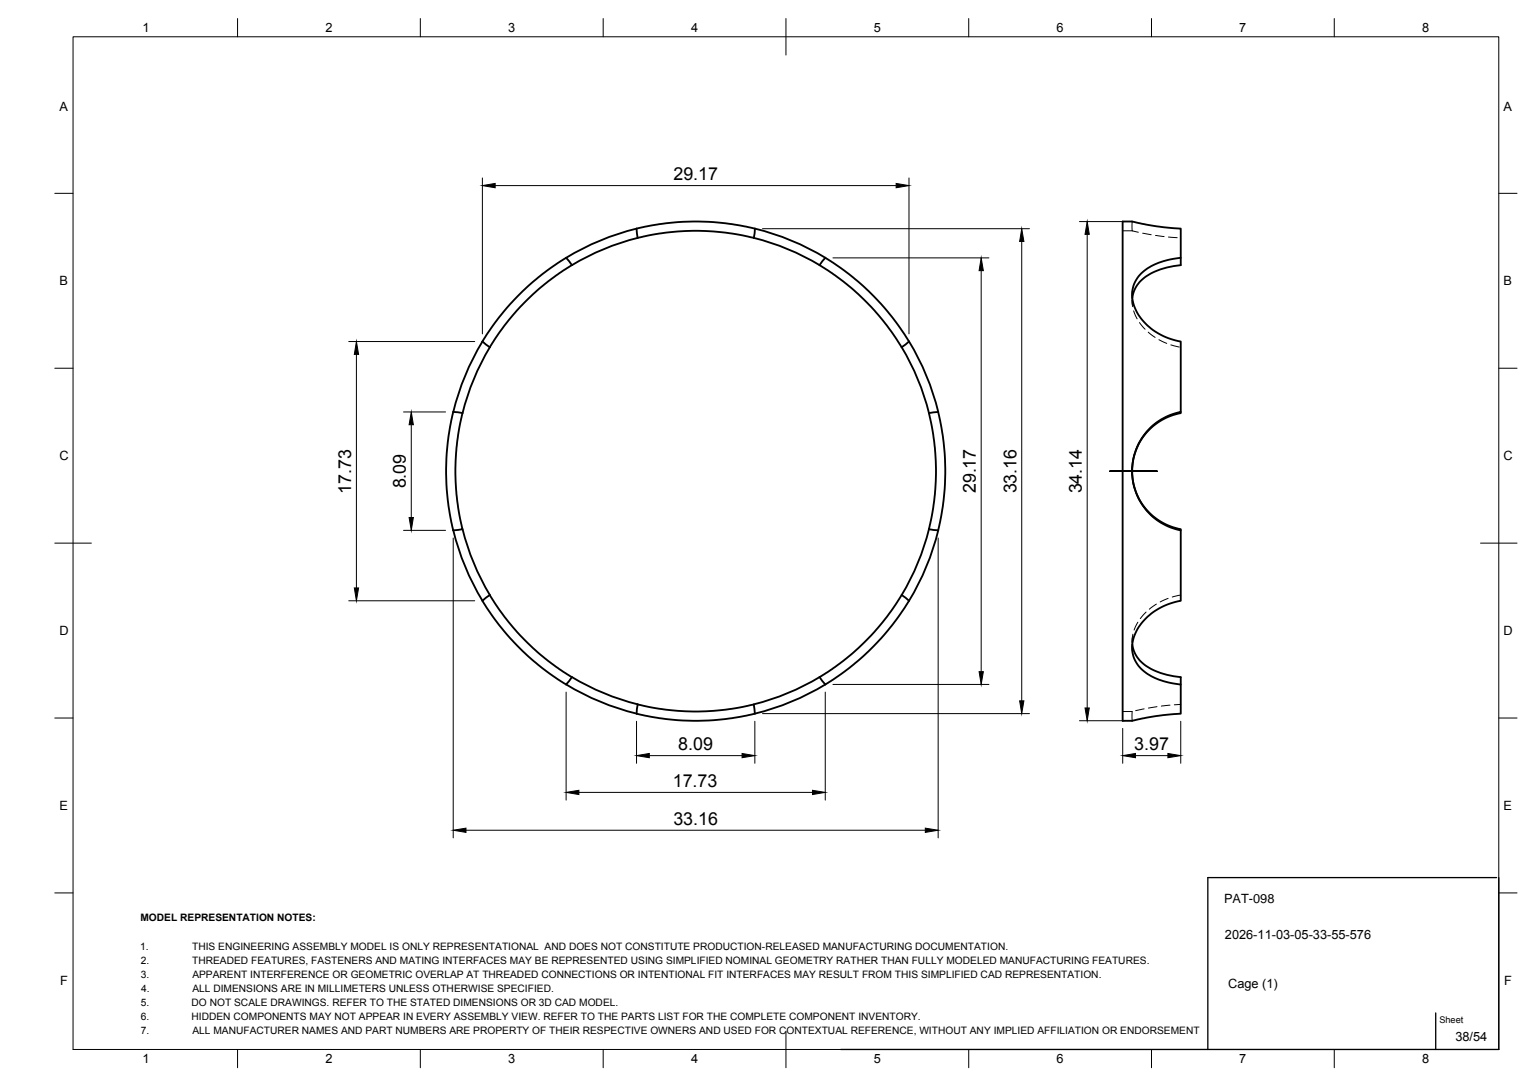
ISO-10303-21;
HEADER;
/* Generated by software containing ST-Developer
 * from STEP Tools, Inc. (www.steptools.com) 
 */

FILE_DESCRIPTION(
/* description */ ('Spring compression tester'),
/* implementation_level */ '2;1');

FILE_NAME(
/* name */ 'Cage (1).step',
/* time_stamp */ '2026-10-28T03:24:11-07:00',
/* author */ (''),
/* organization */ (''),
/* preprocessor_version */ 'ST-DEVELOPER v20.2',
/* originating_system */ 'Autodesk Translation Framework v15.17.0.0',
/* authorisation */ '');

FILE_SCHEMA (('AUTOMOTIVE_DESIGN { 1 0 10303 214 3 1 1 }'));
ENDSEC;

DATA;
#10=MECHANICAL_DESIGN_GEOMETRIC_PRESENTATION_REPRESENTATION('',(#1149),#43521);
#567=B_SPLINE_CURVE_WITH_KNOTS('',3,(#29122,#29123,#29124,#29125,#29126,
#29127,#29128,#29129,#29130,#29131,#29132,#29133,#29134,#29135,#29136,#29137,
#29138,#29139,#29140,#29141,#29142,#29143),.UNSPECIFIED.,.F.,.F.,(4,2,2,
2,2,2,2,2,2,2,4),(0.0789094028588958,0.210573405340968,0.315860108011452,
0.421146810681936,0.522142632548711,0.623138454415485,0.72413427628226,
0.825130098149035,0.930416800819519,1.03570350349,1.16736750597208),
 .UNSPECIFIED.);
#568=B_SPLINE_CURVE_WITH_KNOTS('',3,(#29147,#29148,#29149,#29150,#29151,
#29152,#29153,#29154,#29155,#29156,#29157,#29158,#29159,#29160,#29161,#29162,
#29163,#29164,#29165,#29166,#29167,#29168),.UNSPECIFIED.,.F.,.F.,(4,2,2,
2,2,2,2,2,2,2,4),(0.0774793363974613,0.142088896491891,0.284177792983782,
0.411119756996526,0.514392970548519,0.617666184100513,0.720939397652506,
0.8242126112045,0.951154575217244,1.09324347170913,1.15785303180356),
 .UNSPECIFIED.);
#569=B_SPLINE_CURVE_WITH_KNOTS('',3,(#29174,#29175,#29176,#29177,#29178,
#29179,#29180,#29181,#29182,#29183,#29184,#29185,#29186,#29187,#29188,#29189,
#29190,#29191,#29192,#29193,#29194,#29195),.UNSPECIFIED.,.F.,.F.,(4,2,2,
2,2,2,2,2,2,2,4),(0.0774793363974613,0.142088896491891,0.284177792983782,
0.411119756996525,0.514392970548519,0.617666184100513,0.720939397652506,
0.8242126112045,0.951154575217243,1.09324347170913,1.15785303180356),
 .UNSPECIFIED.);
#570=B_SPLINE_CURVE_WITH_KNOTS('',3,(#29199,#29200,#29201,#29202,#29203,
#29204,#29205,#29206,#29207,#29208,#29209,#29210,#29211,#29212,#29213,#29214,
#29215,#29216,#29217,#29218,#29219,#29220),.UNSPECIFIED.,.F.,.F.,(4,2,2,
2,2,2,2,2,2,2,4),(0.0774793363974614,0.142088896491891,0.284177792983781,
0.411119756996525,0.514392970548519,0.617666184100512,0.720939397652506,
0.824212611204499,0.951154575217243,1.09324347170913,1.15785303180356),
 .UNSPECIFIED.);
#571=B_SPLINE_CURVE_WITH_KNOTS('',3,(#29224,#29225,#29226,#29227,#29228,
#29229,#29230,#29231,#29232,#29233,#29234,#29235),.UNSPECIFIED.,.F.,.F.,
(4,2,2,2,2,4),(0.0774793363974613,0.142088896491891,0.284177792983781,0.411119756996525,
0.514392970548519,0.617666184100512),.UNSPECIFIED.);
#572=B_SPLINE_CURVE_WITH_KNOTS('',3,(#29240,#29241,#29242,#29243,#29244,
#29245,#29246,#29247,#29248,#29249,#29250,#29251),.UNSPECIFIED.,.F.,.F.,
(4,2,2,2,2,4),(0.617666184100512,0.720939397652506,0.824212611204499,0.951154575217243,
1.09324347170913,1.15785303180356),.UNSPECIFIED.);
#573=B_SPLINE_CURVE_WITH_KNOTS('',3,(#29255,#29256,#29257,#29258,#29259,
#29260,#29261,#29262,#29263,#29264,#29265,#29266,#29267,#29268,#29269,#29270,
#29271,#29272,#29273,#29274,#29275,#29276),.UNSPECIFIED.,.F.,.F.,(4,2,2,
2,2,2,2,2,2,2,4),(0.0774793363974613,0.142088896491891,0.284177792983782,
0.411119756996526,0.514392970548519,0.617666184100513,0.720939397652507,
0.8242126112045,0.951154575217245,1.09324347170914,1.15785303180356),
 .UNSPECIFIED.);
#574=B_SPLINE_CURVE_WITH_KNOTS('',3,(#29280,#29281,#29282,#29283,#29284,
#29285,#29286,#29287,#29288,#29289,#29290,#29291,#29292,#29293,#29294,#29295,
#29296,#29297,#29298,#29299,#29300,#29301),.UNSPECIFIED.,.F.,.F.,(4,2,2,
2,2,2,2,2,2,2,4),(0.0774793363974613,0.142088896491891,0.284177792983782,
0.411119756996526,0.514392970548519,0.617666184100513,0.720939397652506,
0.824212611204499,0.951154575217243,1.09324347170913,1.15785303180356),
 .UNSPECIFIED.);
#575=B_SPLINE_CURVE_WITH_KNOTS('',3,(#29305,#29306,#29307,#29308,#29309,
#29310,#29311,#29312,#29313,#29314,#29315,#29316,#29317,#29318,#29319,#29320,
#29321,#29322,#29323,#29324,#29325,#29326),.UNSPECIFIED.,.F.,.F.,(4,2,2,
2,2,2,2,2,2,2,4),(0.0774793363974613,0.142088896491891,0.284177792983782,
0.411119756996526,0.514392970548519,0.617666184100513,0.720939397652506,
0.8242126112045,0.951154575217244,1.09324347170913,1.15785303180356),
 .UNSPECIFIED.);
#576=B_SPLINE_CURVE_WITH_KNOTS('',3,(#29330,#29331,#29332,#29333,#29334,
#29335,#29336,#29337,#29338,#29339,#29340,#29341,#29342,#29343,#29344,#29345,
#29346,#29347,#29348,#29349,#29350,#29351),.UNSPECIFIED.,.F.,.F.,(4,2,2,
2,2,2,2,2,2,2,4),(0.0774793363974613,0.142088896491891,0.284177792983782,
0.411119756996526,0.514392970548519,0.617666184100513,0.720939397652506,
0.8242126112045,0.951154575217243,1.09324347170913,1.15785303180356),
 .UNSPECIFIED.);
#577=B_SPLINE_CURVE_WITH_KNOTS('',3,(#29359,#29360,#29361,#29362,#29363,
#29364,#29365,#29366,#29367,#29368,#29369,#29370,#29371,#29372,#29373,#29374,
#29375,#29376,#29377,#29378,#29379,#29380),.UNSPECIFIED.,.F.,.F.,(4,2,2,
2,2,2,2,2,2,2,4),(0.0789094028588958,0.210573405340968,0.315860108011452,
0.421146810681936,0.522142632548711,0.623138454415485,0.72413427628226,
0.825130098149035,0.930416800819519,1.03570350349,1.16736750597208),
 .UNSPECIFIED.);
#578=B_SPLINE_CURVE_WITH_KNOTS('',3,(#29388,#29389,#29390,#29391,#29392,
#29393,#29394,#29395,#29396,#29397,#29398,#29399,#29400,#29401,#29402,#29403,
#29404,#29405,#29406,#29407,#29408,#29409),.UNSPECIFIED.,.F.,.F.,(4,2,2,
2,2,2,2,2,2,2,4),(0.0789094028588958,0.210573405340969,0.315860108011453,
0.421146810681937,0.522142632548712,0.623138454415486,0.724134276282261,
0.825130098149035,0.930416800819519,1.03570350349,1.16736750597208),
 .UNSPECIFIED.);
#579=B_SPLINE_CURVE_WITH_KNOTS('',3,(#29418,#29419,#29420,#29421,#29422,
#29423,#29424,#29425,#29426,#29427,#29428,#29429),.UNSPECIFIED.,.F.,.F.,
(4,2,2,2,2,4),(0.0789094028588958,0.210573405340968,0.315860108011452,0.421146810681937,
0.522142632548711,0.623138454415486),.UNSPECIFIED.);
#580=B_SPLINE_CURVE_WITH_KNOTS('',3,(#29431,#29432,#29433,#29434,#29435,
#29436,#29437,#29438,#29439,#29440,#29441,#29442),.UNSPECIFIED.,.F.,.F.,
(4,2,2,2,2,4),(0.623138454415486,0.72413427628226,0.825130098149035,0.930416800819519,
1.03570350349,1.16736750597208),.UNSPECIFIED.);
#581=B_SPLINE_CURVE_WITH_KNOTS('',3,(#29449,#29450,#29451,#29452,#29453,
#29454,#29455,#29456,#29457,#29458,#29459,#29460,#29461,#29462,#29463,#29464,
#29465,#29466,#29467,#29468,#29469,#29470),.UNSPECIFIED.,.F.,.F.,(4,2,2,
2,2,2,2,2,2,2,4),(0.0789094028588958,0.210573405340968,0.315860108011452,
0.421146810681936,0.522142632548711,0.623138454415486,0.72413427628226,
0.825130098149035,0.930416800819519,1.03570350349,1.16736750597208),
 .UNSPECIFIED.);
#582=B_SPLINE_CURVE_WITH_KNOTS('',3,(#29478,#29479,#29480,#29481,#29482,
#29483,#29484,#29485,#29486,#29487,#29488,#29489,#29490,#29491,#29492,#29493,
#29494,#29495,#29496,#29497,#29498,#29499),.UNSPECIFIED.,.F.,.F.,(4,2,2,
2,2,2,2,2,2,2,4),(0.0789094028588957,0.210573405340968,0.315860108011452,
0.421146810681936,0.522142632548711,0.623138454415485,0.72413427628226,
0.825130098149035,0.930416800819519,1.03570350349,1.16736750597207),
 .UNSPECIFIED.);
#583=B_SPLINE_CURVE_WITH_KNOTS('',3,(#29507,#29508,#29509,#29510,#29511,
#29512,#29513,#29514,#29515,#29516,#29517,#29518,#29519,#29520,#29521,#29522,
#29523,#29524,#29525,#29526,#29527,#29528),.UNSPECIFIED.,.F.,.F.,(4,2,2,
2,2,2,2,2,2,2,4),(0.0789094028588958,0.210573405340968,0.315860108011452,
0.421146810681936,0.522142632548711,0.623138454415486,0.72413427628226,
0.825130098149035,0.930416800819519,1.03570350349,1.16736750597208),
 .UNSPECIFIED.);
#584=B_SPLINE_CURVE_WITH_KNOTS('',3,(#29537,#29538,#29539,#29540,#29541,
#29542,#29543,#29544,#29545,#29546,#29547,#29548,#29549,#29550,#29551,#29552,
#29553,#29554,#29555,#29556,#29557,#29558),.UNSPECIFIED.,.F.,.F.,(4,2,2,
2,2,2,2,2,2,2,4),(0.0789094028588958,0.210573405340968,0.315860108011452,
0.421146810681936,0.522142632548711,0.623138454415485,0.72413427628226,
0.825130098149035,0.930416800819519,1.03570350349,1.16736750597208),
 .UNSPECIFIED.);
#919=SPHERICAL_SURFACE('',#20179,0.412776);
#920=SPHERICAL_SURFACE('',#20195,0.412776);
#921=SPHERICAL_SURFACE('',#20200,0.412776);
#922=SPHERICAL_SURFACE('',#20205,0.412776);
#923=SPHERICAL_SURFACE('',#20210,0.412776);
#924=SPHERICAL_SURFACE('',#20215,0.412776);
#925=SPHERICAL_SURFACE('',#20220,0.412776);
#926=SPHERICAL_SURFACE('',#20228,0.412776);
#1015=SHAPE_REPRESENTATION_RELATIONSHIP('SRR','None',#43829,#1075);
#1075=ADVANCED_BREP_SHAPE_REPRESENTATION('',(#1223),#43489);
#1149=STYLED_ITEM('',(#44202),#1223);
#1223=MANIFOLD_SOLID_BREP('Continuous crown cage',#18587);
#1463=FACE_BOUND('',#3949,.T.);
#1908=PLANE('',#20192);
#1909=PLANE('',#20197);
#1910=PLANE('',#20202);
#1911=PLANE('',#20207);
#1912=PLANE('',#20212);
#1913=PLANE('',#20217);
#1914=PLANE('',#20226);
#1915=PLANE('',#20230);
#1916=PLANE('',#20231);
#2668=FACE_OUTER_BOUND('',#3931,.T.);
#2669=FACE_OUTER_BOUND('',#3932,.T.);
#2670=FACE_OUTER_BOUND('',#3933,.T.);
#2671=FACE_OUTER_BOUND('',#3934,.T.);
#2672=FACE_OUTER_BOUND('',#3935,.T.);
#2673=FACE_OUTER_BOUND('',#3936,.T.);
#2674=FACE_OUTER_BOUND('',#3937,.T.);
#2675=FACE_OUTER_BOUND('',#3938,.T.);
#2676=FACE_OUTER_BOUND('',#3939,.T.);
#2677=FACE_OUTER_BOUND('',#3940,.T.);
#2678=FACE_OUTER_BOUND('',#3941,.T.);
#2679=FACE_OUTER_BOUND('',#3942,.T.);
#2680=FACE_OUTER_BOUND('',#3943,.T.);
#2681=FACE_OUTER_BOUND('',#3944,.T.);
#2682=FACE_OUTER_BOUND('',#3945,.T.);
#2683=FACE_OUTER_BOUND('',#3946,.T.);
#2684=FACE_OUTER_BOUND('',#3947,.T.);
#2685=FACE_OUTER_BOUND('',#3948,.T.);
#2686=FACE_OUTER_BOUND('',#3950,.T.);
#3931=EDGE_LOOP('',(#14399,#14400,#14401,#14402));
#3932=EDGE_LOOP('',(#14403,#14404,#14405,#14406,#14407,#14408,#14409,#14410,
#14411,#14412,#14413,#14414,#14415,#14416,#14417,#14418,#14419,#14420,#14421,
#14422));
#3933=EDGE_LOOP('',(#14423,#14424,#14425,#14426));
#3934=EDGE_LOOP('',(#14427,#14428,#14429,#14430));
#3935=EDGE_LOOP('',(#14431,#14432,#14433,#14434));
#3936=EDGE_LOOP('',(#14435,#14436,#14437,#14438));
#3937=EDGE_LOOP('',(#14439,#14440,#14441,#14442));
#3938=EDGE_LOOP('',(#14443,#14444,#14445,#14446,#14447,#14448));
#3939=EDGE_LOOP('',(#14449,#14450,#14451,#14452));
#3940=EDGE_LOOP('',(#14453,#14454,#14455,#14456));
#3941=EDGE_LOOP('',(#14457,#14458,#14459,#14460));
#3942=EDGE_LOOP('',(#14461,#14462,#14463,#14464));
#3943=EDGE_LOOP('',(#14465,#14466,#14467,#14468));
#3944=EDGE_LOOP('',(#14469,#14470,#14471,#14472));
#3945=EDGE_LOOP('',(#14473,#14474,#14475,#14476,#14477,#14478,#14479,#14480,
#14481,#14482,#14483,#14484,#14485,#14486,#14487,#14488,#14489,#14490,#14491,
#14492));
#3946=EDGE_LOOP('',(#14493,#14494,#14495,#14496));
#3947=EDGE_LOOP('',(#14497,#14498,#14499,#14500));
#3948=EDGE_LOOP('',(#14501));
#3949=EDGE_LOOP('',(#14502));
#3950=EDGE_LOOP('',(#14503,#14504,#14505,#14506));
#5327=LINE('',#29237,#6759);
#5328=LINE('',#29533,#6760);
#6759=VECTOR('',#23721,1.706752);
#6760=VECTOR('',#23798,1.643248);
#7826=CIRCLE('',#20180,0.405071403305639);
#7827=CIRCLE('',#20181,0.405071403305639);
#7828=CIRCLE('',#20183,1.706752);
#7829=CIRCLE('',#20184,1.706752);
#7830=CIRCLE('',#20185,1.706752);
#7831=CIRCLE('',#20186,1.706752);
#7832=CIRCLE('',#20187,1.706752);
#7833=CIRCLE('',#20188,1.706752);
#7834=CIRCLE('',#20189,1.706752);
#7835=CIRCLE('',#20190,1.706752);
#7836=CIRCLE('',#20191,1.706752);
#7837=CIRCLE('',#20193,1.643248);
#7838=CIRCLE('',#20194,0.405071403305639);
#7839=CIRCLE('',#20196,0.405071403305639);
#7840=CIRCLE('',#20198,1.643248);
#7841=CIRCLE('',#20199,0.405071403305639);
#7842=CIRCLE('',#20201,0.405071403305639);
#7843=CIRCLE('',#20203,1.643248);
#7844=CIRCLE('',#20204,0.405071403305639);
#7845=CIRCLE('',#20206,0.405071403305639);
#7846=CIRCLE('',#20208,1.643248);
#7847=CIRCLE('',#20209,0.405071403305639);
#7848=CIRCLE('',#20211,0.405071403305639);
#7849=CIRCLE('',#20213,1.643248);
#7850=CIRCLE('',#20214,0.405071403305639);
#7851=CIRCLE('',#20216,0.405071403305639);
#7852=CIRCLE('',#20218,1.643248);
#7853=CIRCLE('',#20219,0.405071403305639);
#7854=CIRCLE('',#20221,0.405071403305639);
#7855=CIRCLE('',#20223,1.643248);
#7856=CIRCLE('',#20224,1.643248);
#7857=CIRCLE('',#20225,1.643248);
#7858=CIRCLE('',#20227,0.405071403305639);
#7859=CIRCLE('',#20229,0.405071403305639);
#8879=VERTEX_POINT('',#29120);
#8880=VERTEX_POINT('',#29121);
#8881=VERTEX_POINT('',#29144);
#8882=VERTEX_POINT('',#29146);
#8883=VERTEX_POINT('',#29171);
#8884=VERTEX_POINT('',#29173);
#8885=VERTEX_POINT('',#29196);
#8886=VERTEX_POINT('',#29198);
#8887=VERTEX_POINT('',#29221);
#8888=VERTEX_POINT('',#29223);
#8889=VERTEX_POINT('',#29236);
#8890=VERTEX_POINT('',#29239);
#8891=VERTEX_POINT('',#29252);
#8892=VERTEX_POINT('',#29254);
#8893=VERTEX_POINT('',#29277);
#8894=VERTEX_POINT('',#29279);
#8895=VERTEX_POINT('',#29302);
#8896=VERTEX_POINT('',#29304);
#8897=VERTEX_POINT('',#29327);
#8898=VERTEX_POINT('',#29329);
#8899=VERTEX_POINT('',#29354);
#8900=VERTEX_POINT('',#29358);
#8901=VERTEX_POINT('',#29383);
#8902=VERTEX_POINT('',#29387);
#8903=VERTEX_POINT('',#29412);
#8904=VERTEX_POINT('',#29416);
#8905=VERTEX_POINT('',#29417);
#8906=VERTEX_POINT('',#29444);
#8907=VERTEX_POINT('',#29448);
#8908=VERTEX_POINT('',#29473);
#8909=VERTEX_POINT('',#29477);
#8910=VERTEX_POINT('',#29502);
#8911=VERTEX_POINT('',#29506);
#8912=VERTEX_POINT('',#29531);
#8913=VERTEX_POINT('',#29534);
#8914=VERTEX_POINT('',#29536);
#10864=EDGE_CURVE('',#8879,#8880,#567,.T.);
#10865=EDGE_CURVE('',#8881,#8879,#7826,.T.);
#10866=EDGE_CURVE('',#8882,#8881,#568,.T.);
#10867=EDGE_CURVE('',#8880,#8882,#7827,.T.);
#10868=EDGE_CURVE('',#8883,#8881,#7828,.T.);
#10869=EDGE_CURVE('',#8883,#8884,#569,.T.);
#10870=EDGE_CURVE('',#8885,#8884,#7829,.T.);
#10871=EDGE_CURVE('',#8885,#8886,#570,.T.);
#10872=EDGE_CURVE('',#8887,#8886,#7830,.T.);
#10873=EDGE_CURVE('',#8887,#8888,#571,.T.);
#10874=EDGE_CURVE('',#8888,#8889,#5327,.T.);
#10875=EDGE_CURVE('',#8889,#8889,#7831,.T.);
#10876=EDGE_CURVE('',#8888,#8890,#572,.T.);
#10877=EDGE_CURVE('',#8891,#8890,#7832,.T.);
#10878=EDGE_CURVE('',#8891,#8892,#573,.T.);
#10879=EDGE_CURVE('',#8893,#8892,#7833,.T.);
#10880=EDGE_CURVE('',#8893,#8894,#574,.T.);
#10881=EDGE_CURVE('',#8895,#8894,#7834,.T.);
#10882=EDGE_CURVE('',#8895,#8896,#575,.T.);
#10883=EDGE_CURVE('',#8897,#8896,#7835,.T.);
#10884=EDGE_CURVE('',#8897,#8898,#576,.T.);
#10885=EDGE_CURVE('',#8882,#8898,#7836,.T.);
#10886=EDGE_CURVE('',#8879,#8899,#7837,.T.);
#10887=EDGE_CURVE('',#8899,#8883,#7838,.T.);
#10888=EDGE_CURVE('',#8900,#8899,#577,.T.);
#10889=EDGE_CURVE('',#8884,#8900,#7839,.T.);
#10890=EDGE_CURVE('',#8900,#8901,#7840,.T.);
#10891=EDGE_CURVE('',#8901,#8885,#7841,.T.);
#10892=EDGE_CURVE('',#8902,#8901,#578,.T.);
#10893=EDGE_CURVE('',#8886,#8902,#7842,.T.);
#10894=EDGE_CURVE('',#8902,#8903,#7843,.T.);
#10895=EDGE_CURVE('',#8903,#8887,#7844,.T.);
#10896=EDGE_CURVE('',#8904,#8905,#579,.T.);
#10897=EDGE_CURVE('',#8890,#8904,#7845,.T.);
#10898=EDGE_CURVE('',#8905,#8903,#580,.T.);
#10899=EDGE_CURVE('',#8904,#8906,#7846,.T.);
#10900=EDGE_CURVE('',#8906,#8891,#7847,.T.);
#10901=EDGE_CURVE('',#8907,#8906,#581,.T.);
#10902=EDGE_CURVE('',#8892,#8907,#7848,.T.);
#10903=EDGE_CURVE('',#8907,#8908,#7849,.T.);
#10904=EDGE_CURVE('',#8908,#8893,#7850,.T.);
#10905=EDGE_CURVE('',#8909,#8908,#582,.T.);
#10906=EDGE_CURVE('',#8894,#8909,#7851,.T.);
#10907=EDGE_CURVE('',#8909,#8910,#7852,.T.);
#10908=EDGE_CURVE('',#8910,#8895,#7853,.T.);
#10909=EDGE_CURVE('',#8911,#8910,#583,.T.);
#10910=EDGE_CURVE('',#8896,#8911,#7854,.T.);
#10911=EDGE_CURVE('',#8912,#8912,#7855,.T.);
#10912=EDGE_CURVE('',#8912,#8905,#5328,.T.);
#10913=EDGE_CURVE('',#8913,#8880,#7856,.T.);
#10914=EDGE_CURVE('',#8913,#8914,#584,.T.);
#10915=EDGE_CURVE('',#8911,#8914,#7857,.T.);
#10916=EDGE_CURVE('',#8898,#8913,#7858,.T.);
#10917=EDGE_CURVE('',#8914,#8897,#7859,.T.);
#14399=ORIENTED_EDGE('',*,*,#10864,.F.);
#14400=ORIENTED_EDGE('',*,*,#10865,.F.);
#14401=ORIENTED_EDGE('',*,*,#10866,.F.);
#14402=ORIENTED_EDGE('',*,*,#10867,.F.);
#14403=ORIENTED_EDGE('',*,*,#10866,.T.);
#14404=ORIENTED_EDGE('',*,*,#10868,.F.);
#14405=ORIENTED_EDGE('',*,*,#10869,.T.);
#14406=ORIENTED_EDGE('',*,*,#10870,.F.);
#14407=ORIENTED_EDGE('',*,*,#10871,.T.);
#14408=ORIENTED_EDGE('',*,*,#10872,.F.);
#14409=ORIENTED_EDGE('',*,*,#10873,.T.);
#14410=ORIENTED_EDGE('',*,*,#10874,.T.);
#14411=ORIENTED_EDGE('',*,*,#10875,.F.);
#14412=ORIENTED_EDGE('',*,*,#10874,.F.);
#14413=ORIENTED_EDGE('',*,*,#10876,.T.);
#14414=ORIENTED_EDGE('',*,*,#10877,.F.);
#14415=ORIENTED_EDGE('',*,*,#10878,.T.);
#14416=ORIENTED_EDGE('',*,*,#10879,.F.);
#14417=ORIENTED_EDGE('',*,*,#10880,.T.);
#14418=ORIENTED_EDGE('',*,*,#10881,.F.);
#14419=ORIENTED_EDGE('',*,*,#10882,.T.);
#14420=ORIENTED_EDGE('',*,*,#10883,.F.);
#14421=ORIENTED_EDGE('',*,*,#10884,.T.);
#14422=ORIENTED_EDGE('',*,*,#10885,.F.);
#14423=ORIENTED_EDGE('',*,*,#10865,.T.);
#14424=ORIENTED_EDGE('',*,*,#10886,.T.);
#14425=ORIENTED_EDGE('',*,*,#10887,.T.);
#14426=ORIENTED_EDGE('',*,*,#10868,.T.);
#14427=ORIENTED_EDGE('',*,*,#10888,.F.);
#14428=ORIENTED_EDGE('',*,*,#10889,.F.);
#14429=ORIENTED_EDGE('',*,*,#10869,.F.);
#14430=ORIENTED_EDGE('',*,*,#10887,.F.);
#14431=ORIENTED_EDGE('',*,*,#10889,.T.);
#14432=ORIENTED_EDGE('',*,*,#10890,.T.);
#14433=ORIENTED_EDGE('',*,*,#10891,.T.);
#14434=ORIENTED_EDGE('',*,*,#10870,.T.);
#14435=ORIENTED_EDGE('',*,*,#10892,.F.);
#14436=ORIENTED_EDGE('',*,*,#10893,.F.);
#14437=ORIENTED_EDGE('',*,*,#10871,.F.);
#14438=ORIENTED_EDGE('',*,*,#10891,.F.);
#14439=ORIENTED_EDGE('',*,*,#10893,.T.);
#14440=ORIENTED_EDGE('',*,*,#10894,.T.);
#14441=ORIENTED_EDGE('',*,*,#10895,.T.);
#14442=ORIENTED_EDGE('',*,*,#10872,.T.);
#14443=ORIENTED_EDGE('',*,*,#10896,.F.);
#14444=ORIENTED_EDGE('',*,*,#10897,.F.);
#14445=ORIENTED_EDGE('',*,*,#10876,.F.);
#14446=ORIENTED_EDGE('',*,*,#10873,.F.);
#14447=ORIENTED_EDGE('',*,*,#10895,.F.);
#14448=ORIENTED_EDGE('',*,*,#10898,.F.);
#14449=ORIENTED_EDGE('',*,*,#10897,.T.);
#14450=ORIENTED_EDGE('',*,*,#10899,.T.);
#14451=ORIENTED_EDGE('',*,*,#10900,.T.);
#14452=ORIENTED_EDGE('',*,*,#10877,.T.);
#14453=ORIENTED_EDGE('',*,*,#10901,.F.);
#14454=ORIENTED_EDGE('',*,*,#10902,.F.);
#14455=ORIENTED_EDGE('',*,*,#10878,.F.);
#14456=ORIENTED_EDGE('',*,*,#10900,.F.);
#14457=ORIENTED_EDGE('',*,*,#10902,.T.);
#14458=ORIENTED_EDGE('',*,*,#10903,.T.);
#14459=ORIENTED_EDGE('',*,*,#10904,.T.);
#14460=ORIENTED_EDGE('',*,*,#10879,.T.);
#14461=ORIENTED_EDGE('',*,*,#10905,.F.);
#14462=ORIENTED_EDGE('',*,*,#10906,.F.);
#14463=ORIENTED_EDGE('',*,*,#10880,.F.);
#14464=ORIENTED_EDGE('',*,*,#10904,.F.);
#14465=ORIENTED_EDGE('',*,*,#10906,.T.);
#14466=ORIENTED_EDGE('',*,*,#10907,.T.);
#14467=ORIENTED_EDGE('',*,*,#10908,.T.);
#14468=ORIENTED_EDGE('',*,*,#10881,.T.);
#14469=ORIENTED_EDGE('',*,*,#10882,.F.);
#14470=ORIENTED_EDGE('',*,*,#10908,.F.);
#14471=ORIENTED_EDGE('',*,*,#10909,.F.);
#14472=ORIENTED_EDGE('',*,*,#10910,.F.);
#14473=ORIENTED_EDGE('',*,*,#10911,.F.);
#14474=ORIENTED_EDGE('',*,*,#10912,.T.);
#14475=ORIENTED_EDGE('',*,*,#10898,.T.);
#14476=ORIENTED_EDGE('',*,*,#10894,.F.);
#14477=ORIENTED_EDGE('',*,*,#10892,.T.);
#14478=ORIENTED_EDGE('',*,*,#10890,.F.);
#14479=ORIENTED_EDGE('',*,*,#10888,.T.);
#14480=ORIENTED_EDGE('',*,*,#10886,.F.);
#14481=ORIENTED_EDGE('',*,*,#10864,.T.);
#14482=ORIENTED_EDGE('',*,*,#10913,.F.);
#14483=ORIENTED_EDGE('',*,*,#10914,.T.);
#14484=ORIENTED_EDGE('',*,*,#10915,.F.);
#14485=ORIENTED_EDGE('',*,*,#10909,.T.);
#14486=ORIENTED_EDGE('',*,*,#10907,.F.);
#14487=ORIENTED_EDGE('',*,*,#10905,.T.);
#14488=ORIENTED_EDGE('',*,*,#10903,.F.);
#14489=ORIENTED_EDGE('',*,*,#10901,.T.);
#14490=ORIENTED_EDGE('',*,*,#10899,.F.);
#14491=ORIENTED_EDGE('',*,*,#10896,.T.);
#14492=ORIENTED_EDGE('',*,*,#10912,.F.);
#14493=ORIENTED_EDGE('',*,*,#10867,.T.);
#14494=ORIENTED_EDGE('',*,*,#10885,.T.);
#14495=ORIENTED_EDGE('',*,*,#10916,.T.);
#14496=ORIENTED_EDGE('',*,*,#10913,.T.);
#14497=ORIENTED_EDGE('',*,*,#10884,.F.);
#14498=ORIENTED_EDGE('',*,*,#10917,.F.);
#14499=ORIENTED_EDGE('',*,*,#10914,.F.);
#14500=ORIENTED_EDGE('',*,*,#10916,.F.);
#14501=ORIENTED_EDGE('',*,*,#10875,.T.);
#14502=ORIENTED_EDGE('',*,*,#10911,.T.);
#14503=ORIENTED_EDGE('',*,*,#10910,.T.);
#14504=ORIENTED_EDGE('',*,*,#10915,.T.);
#14505=ORIENTED_EDGE('',*,*,#10917,.T.);
#14506=ORIENTED_EDGE('',*,*,#10883,.T.);
#17245=CYLINDRICAL_SURFACE('',#20182,1.706752);
#17246=CYLINDRICAL_SURFACE('',#20222,1.643248);
#17992=ADVANCED_FACE('',(#2668),#919,.F.);
#17993=ADVANCED_FACE('',(#2669),#17245,.T.);
#17994=ADVANCED_FACE('',(#2670),#1908,.T.);
#17995=ADVANCED_FACE('',(#2671),#920,.F.);
#17996=ADVANCED_FACE('',(#2672),#1909,.T.);
#17997=ADVANCED_FACE('',(#2673),#921,.F.);
#17998=ADVANCED_FACE('',(#2674),#1910,.T.);
#17999=ADVANCED_FACE('',(#2675),#922,.F.);
#18000=ADVANCED_FACE('',(#2676),#1911,.T.);
#18001=ADVANCED_FACE('',(#2677),#923,.F.);
#18002=ADVANCED_FACE('',(#2678),#1912,.T.);
#18003=ADVANCED_FACE('',(#2679),#924,.F.);
#18004=ADVANCED_FACE('',(#2680),#1913,.T.);
#18005=ADVANCED_FACE('',(#2681),#925,.F.);
#18006=ADVANCED_FACE('',(#2682),#17246,.F.);
#18007=ADVANCED_FACE('',(#2683),#1914,.T.);
#18008=ADVANCED_FACE('',(#2684),#926,.F.);
#18009=ADVANCED_FACE('',(#2685,#1463),#1915,.T.);
#18010=ADVANCED_FACE('',(#2686),#1916,.T.);
#18587=CLOSED_SHELL('',(#17992,#17993,#17994,#17995,#17996,#17997,#17998,
#17999,#18000,#18001,#18002,#18003,#18004,#18005,#18006,#18007,#18008,#18009,
#18010));
#20178=AXIS2_PLACEMENT_3D('',#29118,#23705,#23706);
#20179=AXIS2_PLACEMENT_3D('',#29119,#23707,#23708);
#20180=AXIS2_PLACEMENT_3D('',#29145,#23709,#23710);
#20181=AXIS2_PLACEMENT_3D('',#29169,#23711,#23712);
#20182=AXIS2_PLACEMENT_3D('',#29170,#23713,#23714);
#20183=AXIS2_PLACEMENT_3D('',#29172,#23715,#23716);
#20184=AXIS2_PLACEMENT_3D('',#29197,#23717,#23718);
#20185=AXIS2_PLACEMENT_3D('',#29222,#23719,#23720);
#20186=AXIS2_PLACEMENT_3D('',#29238,#23722,#23723);
#20187=AXIS2_PLACEMENT_3D('',#29253,#23724,#23725);
#20188=AXIS2_PLACEMENT_3D('',#29278,#23726,#23727);
#20189=AXIS2_PLACEMENT_3D('',#29303,#23728,#23729);
#20190=AXIS2_PLACEMENT_3D('',#29328,#23730,#23731);
#20191=AXIS2_PLACEMENT_3D('',#29352,#23732,#23733);
#20192=AXIS2_PLACEMENT_3D('',#29353,#23734,#23735);
#20193=AXIS2_PLACEMENT_3D('',#29355,#23736,#23737);
#20194=AXIS2_PLACEMENT_3D('',#29356,#23738,#23739);
#20195=AXIS2_PLACEMENT_3D('',#29357,#23740,#23741);
#20196=AXIS2_PLACEMENT_3D('',#29381,#23742,#23743);
#20197=AXIS2_PLACEMENT_3D('',#29382,#23744,#23745);
#20198=AXIS2_PLACEMENT_3D('',#29384,#23746,#23747);
#20199=AXIS2_PLACEMENT_3D('',#29385,#23748,#23749);
#20200=AXIS2_PLACEMENT_3D('',#29386,#23750,#23751);
#20201=AXIS2_PLACEMENT_3D('',#29410,#23752,#23753);
#20202=AXIS2_PLACEMENT_3D('',#29411,#23754,#23755);
#20203=AXIS2_PLACEMENT_3D('',#29413,#23756,#23757);
#20204=AXIS2_PLACEMENT_3D('',#29414,#23758,#23759);
#20205=AXIS2_PLACEMENT_3D('',#29415,#23760,#23761);
#20206=AXIS2_PLACEMENT_3D('',#29430,#23762,#23763);
#20207=AXIS2_PLACEMENT_3D('',#29443,#23764,#23765);
#20208=AXIS2_PLACEMENT_3D('',#29445,#23766,#23767);
#20209=AXIS2_PLACEMENT_3D('',#29446,#23768,#23769);
#20210=AXIS2_PLACEMENT_3D('',#29447,#23770,#23771);
#20211=AXIS2_PLACEMENT_3D('',#29471,#23772,#23773);
#20212=AXIS2_PLACEMENT_3D('',#29472,#23774,#23775);
#20213=AXIS2_PLACEMENT_3D('',#29474,#23776,#23777);
#20214=AXIS2_PLACEMENT_3D('',#29475,#23778,#23779);
#20215=AXIS2_PLACEMENT_3D('',#29476,#23780,#23781);
#20216=AXIS2_PLACEMENT_3D('',#29500,#23782,#23783);
#20217=AXIS2_PLACEMENT_3D('',#29501,#23784,#23785);
#20218=AXIS2_PLACEMENT_3D('',#29503,#23786,#23787);
#20219=AXIS2_PLACEMENT_3D('',#29504,#23788,#23789);
#20220=AXIS2_PLACEMENT_3D('',#29505,#23790,#23791);
#20221=AXIS2_PLACEMENT_3D('',#29529,#23792,#23793);
#20222=AXIS2_PLACEMENT_3D('',#29530,#23794,#23795);
#20223=AXIS2_PLACEMENT_3D('',#29532,#23796,#23797);
#20224=AXIS2_PLACEMENT_3D('',#29535,#23799,#23800);
#20225=AXIS2_PLACEMENT_3D('',#29559,#23801,#23802);
#20226=AXIS2_PLACEMENT_3D('',#29560,#23803,#23804);
#20227=AXIS2_PLACEMENT_3D('',#29561,#23805,#23806);
#20228=AXIS2_PLACEMENT_3D('',#29562,#23807,#23808);
#20229=AXIS2_PLACEMENT_3D('',#29563,#23809,#23810);
#20230=AXIS2_PLACEMENT_3D('',#29564,#23811,#23812);
#20231=AXIS2_PLACEMENT_3D('',#29565,#23813,#23814);
#23705=DIRECTION('axis',(0.,0.,1.));
#23706=DIRECTION('refdir',(1.,0.,0.));
#23707=DIRECTION('center_axis',(0.,0.,1.));
#23708=DIRECTION('ref_axis',(1.,0.,0.));
#23709=DIRECTION('center_axis',(0.,-1.,0.));
#23710=DIRECTION('ref_axis',(0.,0.,-1.));
#23711=DIRECTION('center_axis',(0.,-1.,0.));
#23712=DIRECTION('ref_axis',(0.,0.,-1.));
#23713=DIRECTION('center_axis',(0.,1.,0.));
#23714=DIRECTION('ref_axis',(1.,0.,0.));
#23715=DIRECTION('center_axis',(0.,1.,0.));
#23716=DIRECTION('ref_axis',(1.,0.,0.));
#23717=DIRECTION('center_axis',(0.,1.,0.));
#23718=DIRECTION('ref_axis',(1.,0.,0.));
#23719=DIRECTION('center_axis',(0.,1.,0.));
#23720=DIRECTION('ref_axis',(1.,0.,0.));
#23721=DIRECTION('',(0.,-1.,0.));
#23722=DIRECTION('center_axis',(0.,-1.,0.));
#23723=DIRECTION('ref_axis',(1.,0.,0.));
#23724=DIRECTION('center_axis',(0.,1.,0.));
#23725=DIRECTION('ref_axis',(1.,0.,0.));
#23726=DIRECTION('center_axis',(0.,1.,0.));
#23727=DIRECTION('ref_axis',(1.,0.,0.));
#23728=DIRECTION('center_axis',(0.,1.,0.));
#23729=DIRECTION('ref_axis',(1.,0.,0.));
#23730=DIRECTION('center_axis',(0.,1.,0.));
#23731=DIRECTION('ref_axis',(1.,0.,0.));
#23732=DIRECTION('center_axis',(0.,1.,0.));
#23733=DIRECTION('ref_axis',(1.,0.,0.));
#23734=DIRECTION('center_axis',(0.,1.,0.));
#23735=DIRECTION('ref_axis',(1.,0.,0.));
#23736=DIRECTION('center_axis',(0.,-1.,0.));
#23737=DIRECTION('ref_axis',(1.,0.,0.));
#23738=DIRECTION('center_axis',(0.,-1.,0.));
#23739=DIRECTION('ref_axis',(0.,0.,-1.));
#23740=DIRECTION('center_axis',(6.12323399573677E-17,0.,1.));
#23741=DIRECTION('ref_axis',(1.,0.,0.));
#23742=DIRECTION('center_axis',(0.,-1.,0.));
#23743=DIRECTION('ref_axis',(0.,0.,-1.));
#23744=DIRECTION('center_axis',(0.,1.,0.));
#23745=DIRECTION('ref_axis',(1.,0.,0.));
#23746=DIRECTION('center_axis',(0.,-1.,0.));
#23747=DIRECTION('ref_axis',(1.,0.,0.));
#23748=DIRECTION('center_axis',(0.,-1.,0.));
#23749=DIRECTION('ref_axis',(0.,0.,-1.));
#23750=DIRECTION('center_axis',(0.,0.,1.));
#23751=DIRECTION('ref_axis',(1.,0.,0.));
#23752=DIRECTION('center_axis',(0.,-1.,0.));
#23753=DIRECTION('ref_axis',(0.,0.,-1.));
#23754=DIRECTION('center_axis',(0.,1.,0.));
#23755=DIRECTION('ref_axis',(1.,0.,0.));
#23756=DIRECTION('center_axis',(0.,-1.,0.));
#23757=DIRECTION('ref_axis',(1.,0.,0.));
#23758=DIRECTION('center_axis',(0.,-1.,0.));
#23759=DIRECTION('ref_axis',(0.,0.,-1.));
#23760=DIRECTION('center_axis',(0.,0.,1.));
#23761=DIRECTION('ref_axis',(1.,0.,0.));
#23762=DIRECTION('center_axis',(0.,-1.,0.));
#23763=DIRECTION('ref_axis',(0.,0.,-1.));
#23764=DIRECTION('center_axis',(0.,1.,0.));
#23765=DIRECTION('ref_axis',(1.,0.,0.));
#23766=DIRECTION('center_axis',(0.,-1.,0.));
#23767=DIRECTION('ref_axis',(1.,0.,0.));
#23768=DIRECTION('center_axis',(0.,-1.,0.));
#23769=DIRECTION('ref_axis',(0.,0.,-1.));
#23770=DIRECTION('center_axis',(0.,0.,1.));
#23771=DIRECTION('ref_axis',(1.,0.,0.));
#23772=DIRECTION('center_axis',(0.,-1.,0.));
#23773=DIRECTION('ref_axis',(0.,0.,-1.));
#23774=DIRECTION('center_axis',(0.,1.,0.));
#23775=DIRECTION('ref_axis',(1.,0.,0.));
#23776=DIRECTION('center_axis',(0.,-1.,0.));
#23777=DIRECTION('ref_axis',(1.,0.,0.));
#23778=DIRECTION('center_axis',(0.,-1.,0.));
#23779=DIRECTION('ref_axis',(0.,0.,-1.));
#23780=DIRECTION('center_axis',(6.12323399573676E-17,0.,1.));
#23781=DIRECTION('ref_axis',(1.,0.,0.));
#23782=DIRECTION('center_axis',(0.,-1.,0.));
#23783=DIRECTION('ref_axis',(0.,0.,-1.));
#23784=DIRECTION('center_axis',(0.,1.,0.));
#23785=DIRECTION('ref_axis',(1.,0.,0.));
#23786=DIRECTION('center_axis',(0.,-1.,0.));
#23787=DIRECTION('ref_axis',(1.,0.,0.));
#23788=DIRECTION('center_axis',(0.,-1.,0.));
#23789=DIRECTION('ref_axis',(0.,0.,-1.));
#23790=DIRECTION('center_axis',(0.,0.,1.));
#23791=DIRECTION('ref_axis',(1.,0.,0.));
#23792=DIRECTION('center_axis',(0.,-1.,0.));
#23793=DIRECTION('ref_axis',(0.,0.,-1.));
#23794=DIRECTION('center_axis',(0.,1.,0.));
#23795=DIRECTION('ref_axis',(1.,0.,0.));
#23796=DIRECTION('center_axis',(0.,1.,0.));
#23797=DIRECTION('ref_axis',(1.,0.,0.));
#23798=DIRECTION('',(0.,1.,0.));
#23799=DIRECTION('center_axis',(0.,-1.,0.));
#23800=DIRECTION('ref_axis',(1.,0.,0.));
#23801=DIRECTION('center_axis',(0.,-1.,0.));
#23802=DIRECTION('ref_axis',(1.,0.,0.));
#23803=DIRECTION('center_axis',(0.,1.,0.));
#23804=DIRECTION('ref_axis',(1.,0.,0.));
#23805=DIRECTION('center_axis',(0.,-1.,0.));
#23806=DIRECTION('ref_axis',(0.,0.,-1.));
#23807=DIRECTION('center_axis',(0.,0.,1.));
#23808=DIRECTION('ref_axis',(1.,0.,0.));
#23809=DIRECTION('center_axis',(0.,-1.,0.));
#23810=DIRECTION('ref_axis',(0.,0.,-1.));
#23811=DIRECTION('center_axis',(0.,-1.,0.));
#23812=DIRECTION('ref_axis',(-1.,0.,0.));
#23813=DIRECTION('center_axis',(0.,1.,0.));
#23814=DIRECTION('ref_axis',(1.,0.,0.));
#29118=CARTESIAN_POINT('',(0.,0.,0.));
#29119=CARTESIAN_POINT('Origin',(1.18440385848747,0.,1.18440385848747));
#29120=CARTESIAN_POINT('',(0.846804978391753,-0.07938,1.40825612658882));
#29121=CARTESIAN_POINT('',(1.40825612658882,-0.07938,0.846804978391754));
#29122=CARTESIAN_POINT('Ctrl Pts',(0.846804978391752,-0.0793800000000001,
1.40825612658882));
#29123=CARTESIAN_POINT('Ctrl Pts',(0.854205272175554,-0.123401821157026,
1.40380622184538));
#29124=CARTESIAN_POINT('Ctrl Pts',(0.867957148219441,-0.166543350814306,
1.39550172959303));
#29125=CARTESIAN_POINT('Ctrl Pts',(0.902193646979982,-0.237231147975234,
1.3735491215176));
#29126=CARTESIAN_POINT('Ctrl Pts',(0.920778333482564,-0.266264900654909,
1.36127834356734));
#29127=CARTESIAN_POINT('Ctrl Pts',(0.962485392528369,-0.317195968905306,
1.33211611256184));
#29128=CARTESIAN_POINT('Ctrl Pts',(0.985600426557816,-0.33909093068465,
1.31521005565926));
#29129=CARTESIAN_POINT('Ctrl Pts',(1.03253285680459,-0.373586846396559,
1.27866649102984));
#29130=CARTESIAN_POINT('Ctrl Pts',(1.05871835910697,-0.388086240756494,
1.25722555095714));
#29131=CARTESIAN_POINT('Ctrl Pts',(1.11153475808518,-0.407068917407805,
1.2107812086231));
#29132=CARTESIAN_POINT('Ctrl Pts',(1.13814686046673,-0.411552957311693,
1.18575674747573));
#29133=CARTESIAN_POINT('Ctrl Pts',(1.18575674747573,-0.411552957311693,
1.13814686046673));
#29134=CARTESIAN_POINT('Ctrl Pts',(1.2107812086231,-0.407068917407805,1.11153475808518));
#29135=CARTESIAN_POINT('Ctrl Pts',(1.25722555095713,-0.388086240756494,
1.05871835910697));
#29136=CARTESIAN_POINT('Ctrl Pts',(1.27866649102984,-0.373586846396559,
1.03253285680459));
#29137=CARTESIAN_POINT('Ctrl Pts',(1.31521005565926,-0.33909093068465,0.985600426557816));
#29138=CARTESIAN_POINT('Ctrl Pts',(1.33211611256184,-0.317195968905306,
0.962485392528369));
#29139=CARTESIAN_POINT('Ctrl Pts',(1.36127834356734,-0.266264900654909,
0.920778333482565));
#29140=CARTESIAN_POINT('Ctrl Pts',(1.3735491215176,-0.237231147975234,0.902193646979983));
#29141=CARTESIAN_POINT('Ctrl Pts',(1.39550172959303,-0.166543350814306,
0.867957148219442));
#29142=CARTESIAN_POINT('Ctrl Pts',(1.40380622184538,-0.123401821157026,
0.854205272175555));
#29143=CARTESIAN_POINT('Ctrl Pts',(1.40825612658882,-0.0793800000000001,
0.846804978391753));
#29144=CARTESIAN_POINT('',(0.886256117232623,-0.07938,1.45861320581289));
#29145=CARTESIAN_POINT('Origin',(1.18440385848747,-0.07938,1.18440385848747));
#29146=CARTESIAN_POINT('',(1.45861320581289,-0.07938,0.886256117232624));
#29147=CARTESIAN_POINT('Ctrl Pts',(1.45861320581289,-0.0793800000000001,
0.886256117232623));
#29148=CARTESIAN_POINT('Ctrl Pts',(1.45630208793976,-0.101649918886749,
0.890059788636852));
#29149=CARTESIAN_POINT('Ctrl Pts',(1.45296717977858,-0.123823518623746,
0.895520212222107));
#29150=CARTESIAN_POINT('Ctrl Pts',(1.43904931717599,-0.192480977588836,
0.917859913453975));
#29151=CARTESIAN_POINT('Ctrl Pts',(1.4243271592157,-0.236152929235938,0.940896403863072));
#29152=CARTESIAN_POINT('Ctrl Pts',(1.39055359345152,-0.303141259068212,
0.990027513266106));
#29153=CARTESIAN_POINT('Ctrl Pts',(1.36743459453896,-0.335108247315849,
1.02199477007745));
#29154=CARTESIAN_POINT('Ctrl Pts',(1.32643091652006,-0.373243761060364,
1.07446535104584));
#29155=CARTESIAN_POINT('Ctrl Pts',(1.30441816675528,-0.387888272594439,
1.10126842659597));
#29156=CARTESIAN_POINT('Ctrl Pts',(1.25681160160691,-0.407041111792943,
1.15530234155453));
#29157=CARTESIAN_POINT('Ctrl Pts',(1.23119764287622,-0.411552957311693,
1.18251418313119));
#29158=CARTESIAN_POINT('Ctrl Pts',(1.18251418313119,-0.411552957311693,
1.23119764287622));
#29159=CARTESIAN_POINT('Ctrl Pts',(1.15530234155453,-0.407041111792943,
1.25681160160691));
#29160=CARTESIAN_POINT('Ctrl Pts',(1.10126842659597,-0.387888272594439,
1.30441816675528));
#29161=CARTESIAN_POINT('Ctrl Pts',(1.07446535104584,-0.373243761060364,
1.32643091652006));
#29162=CARTESIAN_POINT('Ctrl Pts',(1.02199477007745,-0.335108247315848,
1.36743459453896));
#29163=CARTESIAN_POINT('Ctrl Pts',(0.990027513266105,-0.303141259068211,
1.39055359345152));
#29164=CARTESIAN_POINT('Ctrl Pts',(0.940896403863071,-0.236152929235937,
1.42432715921571));
#29165=CARTESIAN_POINT('Ctrl Pts',(0.917859913453974,-0.192480977588835,
1.43904931717599));
#29166=CARTESIAN_POINT('Ctrl Pts',(0.895520212222106,-0.123823518623745,
1.45296717977858));
#29167=CARTESIAN_POINT('Ctrl Pts',(0.890059788636851,-0.101649918886749,
1.45630208793976));
#29168=CARTESIAN_POINT('Ctrl Pts',(0.886256117232622,-0.0793800000000001,
1.45861320581289));
#29169=CARTESIAN_POINT('Origin',(1.18440385848747,-0.07938,1.18440385848747));
#29170=CARTESIAN_POINT('Origin',(0.,-0.27783,0.));
#29171=CARTESIAN_POINT('',(0.404717578595295,-0.07938,1.65807299932179));
#29172=CARTESIAN_POINT('Origin',(0.,-0.07938,0.));
#29173=CARTESIAN_POINT('',(-0.404717578595296,-0.07938,1.65807299932179));
#29174=CARTESIAN_POINT('Ctrl Pts',(0.404717578595296,-0.0793800000000001,
1.65807299932179));
#29175=CARTESIAN_POINT('Ctrl Pts',(0.400393769631747,-0.101649918886749,
1.65912839404491));
#29176=CARTESIAN_POINT('Ctrl Pts',(0.394174530911058,-0.123823518623745,
1.66063136041479));
#29177=CARTESIAN_POINT('Ctrl Pts',(0.368536561654407,-0.192480977588835,
1.66658649961961));
#29178=CARTESIAN_POINT('Ctrl Pts',(0.341837165343982,-0.236152929235937,
1.67246562047521));
#29179=CARTESIAN_POINT('Ctrl Pts',(0.283214707341173,-0.303141259068211,
1.68332504372461));
#29180=CARTESIAN_POINT('Ctrl Pts',(0.244262842368623,-0.335108247315849,
1.68958170688653));
#29181=CARTESIAN_POINT('Ctrl Pts',(0.178166559972324,-0.373243761060364,
1.69769003172132));
#29182=CARTESIAN_POINT('Ctrl Pts',(0.143648558862931,-0.387888272594439,
1.70107730356824));
#29183=CARTESIAN_POINT('Ctrl Pts',(0.0717778861362652,-0.407041111792943,
1.70562212620408));
#29184=CARTESIAN_POINT('Ctrl Pts',(0.0344244045173309,-0.411552957311693,
1.706752));
#29185=CARTESIAN_POINT('Ctrl Pts',(-0.0344244045173315,-0.411552957311693,
1.706752));
#29186=CARTESIAN_POINT('Ctrl Pts',(-0.0717778861362658,-0.407041111792943,
1.70562212620408));
#29187=CARTESIAN_POINT('Ctrl Pts',(-0.143648558862932,-0.387888272594439,
1.70107730356824));
#29188=CARTESIAN_POINT('Ctrl Pts',(-0.178166559972325,-0.373243761060364,
1.69769003172132));
#29189=CARTESIAN_POINT('Ctrl Pts',(-0.244262842368624,-0.335108247315849,
1.68958170688653));
#29190=CARTESIAN_POINT('Ctrl Pts',(-0.283214707341173,-0.303141259068212,
1.68332504372461));
#29191=CARTESIAN_POINT('Ctrl Pts',(-0.341837165343982,-0.236152929235937,
1.67246562047521));
#29192=CARTESIAN_POINT('Ctrl Pts',(-0.368536561654408,-0.192480977588835,
1.66658649961961));
#29193=CARTESIAN_POINT('Ctrl Pts',(-0.394174530911059,-0.123823518623745,
1.66063136041479));
#29194=CARTESIAN_POINT('Ctrl Pts',(-0.400393769631748,-0.101649918886749,
1.65912839404491));
#29195=CARTESIAN_POINT('Ctrl Pts',(-0.404717578595297,-0.0793800000000001,
1.65807299932179));
#29196=CARTESIAN_POINT('',(-0.886256117232624,-0.07938,1.45861320581289));
#29197=CARTESIAN_POINT('Origin',(0.,-0.07938,0.));
#29198=CARTESIAN_POINT('',(-1.45861320581289,-0.07938,0.886256117232623));
#29199=CARTESIAN_POINT('Ctrl Pts',(-0.886256117232623,-0.0793800000000001,
1.45861320581289));
#29200=CARTESIAN_POINT('Ctrl Pts',(-0.890059788636852,-0.101649918886749,
1.45630208793976));
#29201=CARTESIAN_POINT('Ctrl Pts',(-0.895520212222106,-0.123823518623745,
1.45296717977858));
#29202=CARTESIAN_POINT('Ctrl Pts',(-0.917859913453974,-0.192480977588835,
1.43904931717599));
#29203=CARTESIAN_POINT('Ctrl Pts',(-0.940896403863071,-0.236152929235937,
1.4243271592157));
#29204=CARTESIAN_POINT('Ctrl Pts',(-0.990027513266105,-0.303141259068211,
1.39055359345152));
#29205=CARTESIAN_POINT('Ctrl Pts',(-1.02199477007745,-0.335108247315848,
1.36743459453896));
#29206=CARTESIAN_POINT('Ctrl Pts',(-1.07446535104584,-0.373243761060364,
1.32643091652006));
#29207=CARTESIAN_POINT('Ctrl Pts',(-1.10126842659597,-0.387888272594439,
1.30441816675528));
#29208=CARTESIAN_POINT('Ctrl Pts',(-1.15530234155453,-0.407041111792943,
1.25681160160691));
#29209=CARTESIAN_POINT('Ctrl Pts',(-1.18251418313119,-0.411552957311693,
1.23119764287622));
#29210=CARTESIAN_POINT('Ctrl Pts',(-1.23119764287622,-0.411552957311693,
1.18251418313119));
#29211=CARTESIAN_POINT('Ctrl Pts',(-1.25681160160691,-0.407041111792943,
1.15530234155453));
#29212=CARTESIAN_POINT('Ctrl Pts',(-1.30441816675528,-0.387888272594439,
1.10126842659597));
#29213=CARTESIAN_POINT('Ctrl Pts',(-1.32643091652006,-0.373243761060365,
1.07446535104584));
#29214=CARTESIAN_POINT('Ctrl Pts',(-1.36743459453896,-0.335108247315849,
1.02199477007745));
#29215=CARTESIAN_POINT('Ctrl Pts',(-1.39055359345152,-0.303141259068212,
0.990027513266106));
#29216=CARTESIAN_POINT('Ctrl Pts',(-1.4243271592157,-0.236152929235938,
0.940896403863071));
#29217=CARTESIAN_POINT('Ctrl Pts',(-1.43904931717599,-0.192480977588836,
0.917859913453974));
#29218=CARTESIAN_POINT('Ctrl Pts',(-1.45296717977858,-0.123823518623746,
0.895520212222106));
#29219=CARTESIAN_POINT('Ctrl Pts',(-1.45630208793976,-0.101649918886749,
0.890059788636852));
#29220=CARTESIAN_POINT('Ctrl Pts',(-1.45861320581289,-0.0793800000000001,
0.886256117232623));
#29221=CARTESIAN_POINT('',(-1.65807299932179,-0.07938,0.404717578595295));
#29222=CARTESIAN_POINT('Origin',(0.,-0.07938,0.));
#29223=CARTESIAN_POINT('',(-1.706752,-0.411552957311693,2.08591827245526E-16));
#29224=CARTESIAN_POINT('Ctrl Pts',(-1.65807299932179,-0.0793800000000001,
0.404717578595296));
#29225=CARTESIAN_POINT('Ctrl Pts',(-1.65912839404491,-0.101649918886749,
0.400393769631747));
#29226=CARTESIAN_POINT('Ctrl Pts',(-1.66063136041479,-0.123823518623745,
0.394174530911058));
#29227=CARTESIAN_POINT('Ctrl Pts',(-1.66658649961961,-0.192480977588835,
0.368536561654407));
#29228=CARTESIAN_POINT('Ctrl Pts',(-1.67246562047521,-0.236152929235937,
0.341837165343982));
#29229=CARTESIAN_POINT('Ctrl Pts',(-1.68332504372461,-0.303141259068211,
0.283214707341173));
#29230=CARTESIAN_POINT('Ctrl Pts',(-1.68958170688653,-0.335108247315848,
0.244262842368623));
#29231=CARTESIAN_POINT('Ctrl Pts',(-1.69769003172132,-0.373243761060364,
0.178166559972324));
#29232=CARTESIAN_POINT('Ctrl Pts',(-1.70107730356824,-0.387888272594439,
0.143648558862931));
#29233=CARTESIAN_POINT('Ctrl Pts',(-1.70562212620408,-0.407041111792943,
0.0717778861362656));
#29234=CARTESIAN_POINT('Ctrl Pts',(-1.706752,-0.411552957311693,0.0344244045173313));
#29235=CARTESIAN_POINT('Ctrl Pts',(-1.706752,-0.411552957311693,2.08166817117217E-16));
#29236=CARTESIAN_POINT('',(-1.706752,-0.47628,2.09016837373834E-16));
#29237=CARTESIAN_POINT('',(-1.706752,-0.27783,2.09016837373834E-16));
#29238=CARTESIAN_POINT('Origin',(0.,-0.47628,0.));
#29239=CARTESIAN_POINT('',(-1.65807299932179,-0.07938,-0.404717578595296));
#29240=CARTESIAN_POINT('Ctrl Pts',(-1.706752,-0.411552957311693,2.0122792321331E-16));
#29241=CARTESIAN_POINT('Ctrl Pts',(-1.706752,-0.411552957311693,-0.0344244045173309));
#29242=CARTESIAN_POINT('Ctrl Pts',(-1.70562212620408,-0.407041111792943,
-0.0717778861362652));
#29243=CARTESIAN_POINT('Ctrl Pts',(-1.70107730356824,-0.387888272594439,
-0.143648558862931));
#29244=CARTESIAN_POINT('Ctrl Pts',(-1.69769003172132,-0.373243761060365,
-0.178166559972324));
#29245=CARTESIAN_POINT('Ctrl Pts',(-1.68958170688653,-0.335108247315849,
-0.244262842368623));
#29246=CARTESIAN_POINT('Ctrl Pts',(-1.68332504372461,-0.303141259068212,
-0.283214707341173));
#29247=CARTESIAN_POINT('Ctrl Pts',(-1.67246562047521,-0.236152929235938,
-0.341837165343982));
#29248=CARTESIAN_POINT('Ctrl Pts',(-1.66658649961961,-0.192480977588836,
-0.368536561654407));
#29249=CARTESIAN_POINT('Ctrl Pts',(-1.66063136041479,-0.123823518623745,
-0.394174530911059));
#29250=CARTESIAN_POINT('Ctrl Pts',(-1.65912839404491,-0.101649918886749,
-0.400393769631748));
#29251=CARTESIAN_POINT('Ctrl Pts',(-1.65807299932179,-0.0793800000000001,
-0.404717578595296));
#29252=CARTESIAN_POINT('',(-1.45861320581289,-0.07938,-0.886256117232623));
#29253=CARTESIAN_POINT('Origin',(0.,-0.07938,0.));
#29254=CARTESIAN_POINT('',(-0.886256117232623,-0.07938,-1.45861320581289));
#29255=CARTESIAN_POINT('Ctrl Pts',(-1.45861320581289,-0.0793800000000001,
-0.886256117232623));
#29256=CARTESIAN_POINT('Ctrl Pts',(-1.45630208793976,-0.101649918886749,
-0.890059788636852));
#29257=CARTESIAN_POINT('Ctrl Pts',(-1.45296717977858,-0.123823518623745,
-0.895520212222106));
#29258=CARTESIAN_POINT('Ctrl Pts',(-1.43904931717599,-0.192480977588835,
-0.917859913453974));
#29259=CARTESIAN_POINT('Ctrl Pts',(-1.4243271592157,-0.236152929235937,
-0.940896403863072));
#29260=CARTESIAN_POINT('Ctrl Pts',(-1.39055359345152,-0.303141259068212,
-0.990027513266106));
#29261=CARTESIAN_POINT('Ctrl Pts',(-1.36743459453896,-0.335108247315849,
-1.02199477007745));
#29262=CARTESIAN_POINT('Ctrl Pts',(-1.32643091652006,-0.373243761060364,
-1.07446535104584));
#29263=CARTESIAN_POINT('Ctrl Pts',(-1.30441816675528,-0.387888272594439,
-1.10126842659597));
#29264=CARTESIAN_POINT('Ctrl Pts',(-1.25681160160691,-0.407041111792943,
-1.15530234155453));
#29265=CARTESIAN_POINT('Ctrl Pts',(-1.23119764287622,-0.411552957311693,
-1.18251418313119));
#29266=CARTESIAN_POINT('Ctrl Pts',(-1.18251418313119,-0.411552957311693,
-1.23119764287622));
#29267=CARTESIAN_POINT('Ctrl Pts',(-1.15530234155453,-0.407041111792943,
-1.25681160160691));
#29268=CARTESIAN_POINT('Ctrl Pts',(-1.10126842659597,-0.387888272594439,
-1.30441816675528));
#29269=CARTESIAN_POINT('Ctrl Pts',(-1.07446535104584,-0.373243761060364,
-1.32643091652006));
#29270=CARTESIAN_POINT('Ctrl Pts',(-1.02199477007745,-0.335108247315848,
-1.36743459453896));
#29271=CARTESIAN_POINT('Ctrl Pts',(-0.990027513266105,-0.303141259068211,
-1.39055359345152));
#29272=CARTESIAN_POINT('Ctrl Pts',(-0.940896403863071,-0.236152929235936,
-1.42432715921571));
#29273=CARTESIAN_POINT('Ctrl Pts',(-0.917859913453974,-0.192480977588835,
-1.43904931717599));
#29274=CARTESIAN_POINT('Ctrl Pts',(-0.895520212222106,-0.123823518623745,
-1.45296717977858));
#29275=CARTESIAN_POINT('Ctrl Pts',(-0.890059788636851,-0.101649918886749,
-1.45630208793976));
#29276=CARTESIAN_POINT('Ctrl Pts',(-0.886256117232623,-0.0793800000000001,
-1.45861320581289));
#29277=CARTESIAN_POINT('',(-0.404717578595295,-0.07938,-1.65807299932179));
#29278=CARTESIAN_POINT('Origin',(0.,-0.07938,0.));
#29279=CARTESIAN_POINT('',(0.404717578595296,-0.07938,-1.65807299932179));
#29280=CARTESIAN_POINT('Ctrl Pts',(-0.404717578595296,-0.0793800000000001,
-1.65807299932179));
#29281=CARTESIAN_POINT('Ctrl Pts',(-0.400393769631747,-0.101649918886749,
-1.65912839404491));
#29282=CARTESIAN_POINT('Ctrl Pts',(-0.394174530911058,-0.123823518623746,
-1.66063136041479));
#29283=CARTESIAN_POINT('Ctrl Pts',(-0.368536561654407,-0.192480977588836,
-1.66658649961961));
#29284=CARTESIAN_POINT('Ctrl Pts',(-0.341837165343982,-0.236152929235938,
-1.67246562047521));
#29285=CARTESIAN_POINT('Ctrl Pts',(-0.283214707341173,-0.303141259068212,
-1.68332504372461));
#29286=CARTESIAN_POINT('Ctrl Pts',(-0.244262842368623,-0.335108247315849,
-1.68958170688653));
#29287=CARTESIAN_POINT('Ctrl Pts',(-0.178166559972324,-0.373243761060364,
-1.69769003172132));
#29288=CARTESIAN_POINT('Ctrl Pts',(-0.143648558862931,-0.387888272594439,
-1.70107730356824));
#29289=CARTESIAN_POINT('Ctrl Pts',(-0.0717778861362653,-0.407041111792943,
-1.70562212620408));
#29290=CARTESIAN_POINT('Ctrl Pts',(-0.034424404517331,-0.411552957311693,
-1.706752));
#29291=CARTESIAN_POINT('Ctrl Pts',(0.0344244045173312,-0.411552957311693,
-1.706752));
#29292=CARTESIAN_POINT('Ctrl Pts',(0.0717778861362655,-0.407041111792943,
-1.70562212620408));
#29293=CARTESIAN_POINT('Ctrl Pts',(0.143648558862931,-0.387888272594439,
-1.70107730356824));
#29294=CARTESIAN_POINT('Ctrl Pts',(0.178166559972324,-0.373243761060364,
-1.69769003172132));
#29295=CARTESIAN_POINT('Ctrl Pts',(0.244262842368623,-0.335108247315849,
-1.68958170688653));
#29296=CARTESIAN_POINT('Ctrl Pts',(0.283214707341173,-0.303141259068212,
-1.68332504372461));
#29297=CARTESIAN_POINT('Ctrl Pts',(0.341837165343982,-0.236152929235937,
-1.67246562047521));
#29298=CARTESIAN_POINT('Ctrl Pts',(0.368536561654407,-0.192480977588835,
-1.66658649961961));
#29299=CARTESIAN_POINT('Ctrl Pts',(0.394174530911059,-0.123823518623745,
-1.66063136041479));
#29300=CARTESIAN_POINT('Ctrl Pts',(0.400393769631748,-0.101649918886749,
-1.65912839404491));
#29301=CARTESIAN_POINT('Ctrl Pts',(0.404717578595296,-0.0793800000000001,
-1.65807299932179));
#29302=CARTESIAN_POINT('',(0.886256117232623,-0.07938,-1.45861320581289));
#29303=CARTESIAN_POINT('Origin',(0.,-0.07938,0.));
#29304=CARTESIAN_POINT('',(1.45861320581289,-0.07938,-0.886256117232623));
#29305=CARTESIAN_POINT('Ctrl Pts',(0.886256117232623,-0.0793800000000001,
-1.45861320581289));
#29306=CARTESIAN_POINT('Ctrl Pts',(0.890059788636852,-0.101649918886749,
-1.45630208793976));
#29307=CARTESIAN_POINT('Ctrl Pts',(0.895520212222106,-0.123823518623745,
-1.45296717977858));
#29308=CARTESIAN_POINT('Ctrl Pts',(0.917859913453974,-0.192480977588835,
-1.43904931717599));
#29309=CARTESIAN_POINT('Ctrl Pts',(0.940896403863072,-0.236152929235937,
-1.4243271592157));
#29310=CARTESIAN_POINT('Ctrl Pts',(0.990027513266106,-0.303141259068211,
-1.39055359345152));
#29311=CARTESIAN_POINT('Ctrl Pts',(1.02199477007745,-0.335108247315849,
-1.36743459453896));
#29312=CARTESIAN_POINT('Ctrl Pts',(1.07446535104584,-0.373243761060364,
-1.32643091652006));
#29313=CARTESIAN_POINT('Ctrl Pts',(1.10126842659597,-0.387888272594439,
-1.30441816675528));
#29314=CARTESIAN_POINT('Ctrl Pts',(1.15530234155453,-0.407041111792943,
-1.25681160160691));
#29315=CARTESIAN_POINT('Ctrl Pts',(1.18251418313119,-0.411552957311693,
-1.23119764287622));
#29316=CARTESIAN_POINT('Ctrl Pts',(1.23119764287622,-0.411552957311693,
-1.18251418313119));
#29317=CARTESIAN_POINT('Ctrl Pts',(1.25681160160691,-0.407041111792943,
-1.15530234155453));
#29318=CARTESIAN_POINT('Ctrl Pts',(1.30441816675528,-0.387888272594439,
-1.10126842659597));
#29319=CARTESIAN_POINT('Ctrl Pts',(1.32643091652006,-0.373243761060364,
-1.07446535104584));
#29320=CARTESIAN_POINT('Ctrl Pts',(1.36743459453896,-0.335108247315849,
-1.02199477007745));
#29321=CARTESIAN_POINT('Ctrl Pts',(1.39055359345152,-0.303141259068212,
-0.990027513266105));
#29322=CARTESIAN_POINT('Ctrl Pts',(1.4243271592157,-0.236152929235937,-0.940896403863071));
#29323=CARTESIAN_POINT('Ctrl Pts',(1.43904931717599,-0.192480977588835,
-0.917859913453974));
#29324=CARTESIAN_POINT('Ctrl Pts',(1.45296717977858,-0.123823518623745,
-0.895520212222106));
#29325=CARTESIAN_POINT('Ctrl Pts',(1.45630208793976,-0.101649918886749,
-0.890059788636852));
#29326=CARTESIAN_POINT('Ctrl Pts',(1.45861320581289,-0.0793800000000001,
-0.886256117232623));
#29327=CARTESIAN_POINT('',(1.65807299932179,-0.07938,-0.404717578595296));
#29328=CARTESIAN_POINT('Origin',(0.,-0.07938,0.));
#29329=CARTESIAN_POINT('',(1.65807299932179,-0.07938,0.404717578595296));
#29330=CARTESIAN_POINT('Ctrl Pts',(1.65807299932179,-0.0793800000000001,
-0.404717578595296));
#29331=CARTESIAN_POINT('Ctrl Pts',(1.65912839404491,-0.101649918886749,
-0.400393769631747));
#29332=CARTESIAN_POINT('Ctrl Pts',(1.66063136041479,-0.123823518623745,
-0.394174530911058));
#29333=CARTESIAN_POINT('Ctrl Pts',(1.66658649961961,-0.192480977588835,
-0.368536561654407));
#29334=CARTESIAN_POINT('Ctrl Pts',(1.67246562047521,-0.236152929235937,
-0.341837165343982));
#29335=CARTESIAN_POINT('Ctrl Pts',(1.68332504372461,-0.303141259068212,
-0.283214707341173));
#29336=CARTESIAN_POINT('Ctrl Pts',(1.68958170688653,-0.335108247315849,
-0.244262842368623));
#29337=CARTESIAN_POINT('Ctrl Pts',(1.69769003172132,-0.373243761060364,
-0.178166559972324));
#29338=CARTESIAN_POINT('Ctrl Pts',(1.70107730356824,-0.387888272594439,
-0.143648558862931));
#29339=CARTESIAN_POINT('Ctrl Pts',(1.70562212620408,-0.407041111792943,
-0.0717778861362655));
#29340=CARTESIAN_POINT('Ctrl Pts',(1.706752,-0.411552957311693,-0.0344244045173312));
#29341=CARTESIAN_POINT('Ctrl Pts',(1.706752,-0.411552957311693,0.0344244045173312));
#29342=CARTESIAN_POINT('Ctrl Pts',(1.70562212620408,-0.407041111792943,
0.0717778861362655));
#29343=CARTESIAN_POINT('Ctrl Pts',(1.70107730356824,-0.387888272594439,
0.143648558862931));
#29344=CARTESIAN_POINT('Ctrl Pts',(1.69769003172132,-0.373243761060364,
0.178166559972324));
#29345=CARTESIAN_POINT('Ctrl Pts',(1.68958170688653,-0.335108247315849,
0.244262842368623));
#29346=CARTESIAN_POINT('Ctrl Pts',(1.68332504372461,-0.303141259068212,
0.283214707341173));
#29347=CARTESIAN_POINT('Ctrl Pts',(1.67246562047521,-0.236152929235937,
0.341837165343982));
#29348=CARTESIAN_POINT('Ctrl Pts',(1.66658649961961,-0.192480977588835,
0.368536561654407));
#29349=CARTESIAN_POINT('Ctrl Pts',(1.66063136041479,-0.123823518623745,
0.394174530911058));
#29350=CARTESIAN_POINT('Ctrl Pts',(1.65912839404491,-0.101649918886749,
0.400393769631747));
#29351=CARTESIAN_POINT('Ctrl Pts',(1.65807299932179,-0.0793800000000001,
0.404717578595296));
#29352=CARTESIAN_POINT('Origin',(0.,-0.07938,0.));
#29353=CARTESIAN_POINT('Origin',(0.,-0.07938,0.));
#29354=CARTESIAN_POINT('',(0.397005914195118,-0.07938,1.59456899932179));
#29355=CARTESIAN_POINT('Origin',(0.,-0.07938,0.));
#29356=CARTESIAN_POINT('Origin',(-3.33066907387547E-16,-0.07938,1.675));
#29357=CARTESIAN_POINT('Origin',(-3.33066907387547E-16,0.,1.675));
#29358=CARTESIAN_POINT('',(-0.397005914195118,-0.07938,1.59456899932179));
#29359=CARTESIAN_POINT('Ctrl Pts',(-0.397005914195119,-0.0793800000000001,
1.59456899932179));
#29360=CARTESIAN_POINT('Ctrl Pts',(-0.3886265584581,-0.123401821157026,
1.59665523941937));
#29361=CARTESIAN_POINT('Ctrl Pts',(-0.373030350867485,-0.166543350814306,
1.60050712143809));
#29362=CARTESIAN_POINT('Ctrl Pts',(-0.333298652394954,-0.237231147975234,
1.60919314384089));
#29363=CARTESIAN_POINT('Ctrl Pts',(-0.311480544243687,-0.266264900654909,
1.61365775139403));
#29364=CARTESIAN_POINT('Ctrl Pts',(-0.261368388670537,-0.317195968905306,
1.62252828437015));
#29365=CARTESIAN_POINT('Ctrl Pts',(-0.233069203882014,-0.33909093068465,
1.62691869420078));
#29366=CARTESIAN_POINT('Ctrl Pts',(-0.174042761838764,-0.373586846396559,
1.63426473152765));
#29367=CARTESIAN_POINT('Ctrl Pts',(-0.14036578147155,-0.388086240756494,
1.63761964365402));
#29368=CARTESIAN_POINT('Ctrl Pts',(-0.0701778381840615,-0.407068917407805,
1.64212536811722));
#29369=CARTESIAN_POINT('Ctrl Pts',(-0.0336652739555918,-0.411552957311693,
1.643248));
#29370=CARTESIAN_POINT('Ctrl Pts',(0.0336652739555913,-0.411552957311693,
1.643248));
#29371=CARTESIAN_POINT('Ctrl Pts',(0.070177838184061,-0.407068917407805,
1.64212536811722));
#29372=CARTESIAN_POINT('Ctrl Pts',(0.140365781471549,-0.388086240756494,
1.63761964365402));
#29373=CARTESIAN_POINT('Ctrl Pts',(0.174042761838763,-0.373586846396559,
1.63426473152765));
#29374=CARTESIAN_POINT('Ctrl Pts',(0.233069203882014,-0.33909093068465,
1.62691869420078));
#29375=CARTESIAN_POINT('Ctrl Pts',(0.261368388670536,-0.317195968905306,
1.62252828437015));
#29376=CARTESIAN_POINT('Ctrl Pts',(0.311480544243686,-0.266264900654908,
1.61365775139403));
#29377=CARTESIAN_POINT('Ctrl Pts',(0.333298652394954,-0.237231147975234,
1.60919314384089));
#29378=CARTESIAN_POINT('Ctrl Pts',(0.373030350867484,-0.166543350814306,
1.60050712143809));
#29379=CARTESIAN_POINT('Ctrl Pts',(0.388626558458099,-0.123401821157026,
1.59665523941937));
#29380=CARTESIAN_POINT('Ctrl Pts',(0.397005914195118,-0.07938,1.59456899932179));
#29381=CARTESIAN_POINT('Origin',(-3.33066907387547E-16,-0.07938,1.675));
#29382=CARTESIAN_POINT('Origin',(0.,-0.07938,0.));
#29383=CARTESIAN_POINT('',(-0.846804978391754,-0.07938,1.40825612658882));
#29384=CARTESIAN_POINT('Origin',(0.,-0.07938,0.));
#29385=CARTESIAN_POINT('Origin',(-1.18440385848747,-0.07938,1.18440385848747));
#29386=CARTESIAN_POINT('Origin',(-1.18440385848747,0.,1.18440385848747));
#29387=CARTESIAN_POINT('',(-1.40825612658882,-0.07938,0.846804978391753));
#29388=CARTESIAN_POINT('Ctrl Pts',(-1.40825612658882,-0.0793800000000001,
0.846804978391753));
#29389=CARTESIAN_POINT('Ctrl Pts',(-1.40380622184538,-0.123401821157026,
0.854205272175555));
#29390=CARTESIAN_POINT('Ctrl Pts',(-1.39550172959303,-0.166543350814306,
0.867957148219442));
#29391=CARTESIAN_POINT('Ctrl Pts',(-1.3735491215176,-0.237231147975235,
0.902193646979983));
#29392=CARTESIAN_POINT('Ctrl Pts',(-1.36127834356734,-0.266264900654909,
0.920778333482565));
#29393=CARTESIAN_POINT('Ctrl Pts',(-1.33211611256184,-0.317195968905306,
0.962485392528369));
#29394=CARTESIAN_POINT('Ctrl Pts',(-1.31521005565926,-0.339090930684651,
0.985600426557816));
#29395=CARTESIAN_POINT('Ctrl Pts',(-1.27866649102984,-0.373586846396559,
1.03253285680459));
#29396=CARTESIAN_POINT('Ctrl Pts',(-1.25722555095714,-0.388086240756494,
1.05871835910697));
#29397=CARTESIAN_POINT('Ctrl Pts',(-1.2107812086231,-0.407068917407805,
1.11153475808518));
#29398=CARTESIAN_POINT('Ctrl Pts',(-1.18575674747573,-0.411552957311693,
1.13814686046673));
#29399=CARTESIAN_POINT('Ctrl Pts',(-1.13814686046673,-0.411552957311693,
1.18575674747573));
#29400=CARTESIAN_POINT('Ctrl Pts',(-1.11153475808518,-0.407068917407805,
1.2107812086231));
#29401=CARTESIAN_POINT('Ctrl Pts',(-1.05871835910697,-0.388086240756494,
1.25722555095714));
#29402=CARTESIAN_POINT('Ctrl Pts',(-1.03253285680459,-0.373586846396559,
1.27866649102984));
#29403=CARTESIAN_POINT('Ctrl Pts',(-0.985600426557816,-0.33909093068465,
1.31521005565926));
#29404=CARTESIAN_POINT('Ctrl Pts',(-0.962485392528369,-0.317195968905306,
1.33211611256184));
#29405=CARTESIAN_POINT('Ctrl Pts',(-0.920778333482565,-0.266264900654908,
1.36127834356734));
#29406=CARTESIAN_POINT('Ctrl Pts',(-0.902193646979983,-0.237231147975234,
1.3735491215176));
#29407=CARTESIAN_POINT('Ctrl Pts',(-0.867957148219442,-0.166543350814306,
1.39550172959303));
#29408=CARTESIAN_POINT('Ctrl Pts',(-0.854205272175555,-0.123401821157026,
1.40380622184538));
#29409=CARTESIAN_POINT('Ctrl Pts',(-0.846804978391753,-0.0793800000000001,
1.40825612658882));
#29410=CARTESIAN_POINT('Origin',(-1.18440385848747,-0.07938,1.18440385848747));
#29411=CARTESIAN_POINT('Origin',(0.,-0.07938,0.));
#29412=CARTESIAN_POINT('',(-1.59456899932179,-0.07938,0.397005914195118));
#29413=CARTESIAN_POINT('Origin',(0.,-0.07938,0.));
#29414=CARTESIAN_POINT('Origin',(-1.675,-0.07938,-2.22044604925031E-16));
#29415=CARTESIAN_POINT('Origin',(-1.675,0.,-2.22044604925031E-16));
#29416=CARTESIAN_POINT('',(-1.59456899932179,-0.07938,-0.397005914195118));
#29417=CARTESIAN_POINT('',(-1.643248,-0.411552957311693,3.47540551556327E-18));
#29418=CARTESIAN_POINT('Ctrl Pts',(-1.59456899932179,-0.0793800000000001,
-0.397005914195119));
#29419=CARTESIAN_POINT('Ctrl Pts',(-1.59665523941937,-0.123401821157026,
-0.388626558458099));
#29420=CARTESIAN_POINT('Ctrl Pts',(-1.60050712143809,-0.166543350814306,
-0.373030350867485));
#29421=CARTESIAN_POINT('Ctrl Pts',(-1.60919314384089,-0.237231147975234,
-0.333298652394954));
#29422=CARTESIAN_POINT('Ctrl Pts',(-1.61365775139403,-0.266264900654909,
-0.311480544243686));
#29423=CARTESIAN_POINT('Ctrl Pts',(-1.62252828437015,-0.317195968905306,
-0.261368388670537));
#29424=CARTESIAN_POINT('Ctrl Pts',(-1.62691869420078,-0.33909093068465,
-0.233069203882014));
#29425=CARTESIAN_POINT('Ctrl Pts',(-1.63426473152765,-0.373586846396559,
-0.174042761838764));
#29426=CARTESIAN_POINT('Ctrl Pts',(-1.63761964365402,-0.388086240756494,
-0.140365781471549));
#29427=CARTESIAN_POINT('Ctrl Pts',(-1.64212536811722,-0.407068917407805,
-0.0701778381840614));
#29428=CARTESIAN_POINT('Ctrl Pts',(-1.643248,-0.411552957311693,-0.0336652739555917));
#29429=CARTESIAN_POINT('Ctrl Pts',(-1.643248,-0.411552957311693,-2.0122792321331E-16));
#29430=CARTESIAN_POINT('Origin',(-1.675,-0.07938,-2.22044604925031E-16));
#29431=CARTESIAN_POINT('Ctrl Pts',(-1.643248,-0.411552957311693,-1.94289029309402E-16));
#29432=CARTESIAN_POINT('Ctrl Pts',(-1.643248,-0.411552957311693,0.0336652739555913));
#29433=CARTESIAN_POINT('Ctrl Pts',(-1.64212536811722,-0.407068917407805,
0.0701778381840609));
#29434=CARTESIAN_POINT('Ctrl Pts',(-1.63761964365402,-0.388086240756494,
0.140365781471549));
#29435=CARTESIAN_POINT('Ctrl Pts',(-1.63426473152765,-0.373586846396559,
0.174042761838763));
#29436=CARTESIAN_POINT('Ctrl Pts',(-1.62691869420078,-0.33909093068465,
0.233069203882014));
#29437=CARTESIAN_POINT('Ctrl Pts',(-1.62252828437015,-0.317195968905306,
0.261368388670536));
#29438=CARTESIAN_POINT('Ctrl Pts',(-1.61365775139403,-0.266264900654909,
0.311480544243686));
#29439=CARTESIAN_POINT('Ctrl Pts',(-1.60919314384089,-0.237231147975235,
0.333298652394954));
#29440=CARTESIAN_POINT('Ctrl Pts',(-1.60050712143809,-0.166543350814306,
0.373030350867484));
#29441=CARTESIAN_POINT('Ctrl Pts',(-1.59665523941937,-0.123401821157026,
0.388626558458099));
#29442=CARTESIAN_POINT('Ctrl Pts',(-1.59456899932179,-0.0793800000000001,
0.397005914195118));
#29443=CARTESIAN_POINT('Origin',(0.,-0.07938,0.));
#29444=CARTESIAN_POINT('',(-1.40825612658882,-0.07938,-0.846804978391753));
#29445=CARTESIAN_POINT('Origin',(0.,-0.07938,0.));
#29446=CARTESIAN_POINT('Origin',(-1.18440385848747,-0.07938,-1.18440385848747));
#29447=CARTESIAN_POINT('Origin',(-1.18440385848747,0.,-1.18440385848747));
#29448=CARTESIAN_POINT('',(-0.846804978391753,-0.07938,-1.40825612658882));
#29449=CARTESIAN_POINT('Ctrl Pts',(-0.846804978391753,-0.0793800000000001,
-1.40825612658882));
#29450=CARTESIAN_POINT('Ctrl Pts',(-0.854205272175555,-0.123401821157026,
-1.40380622184538));
#29451=CARTESIAN_POINT('Ctrl Pts',(-0.867957148219442,-0.166543350814306,
-1.39550172959303));
#29452=CARTESIAN_POINT('Ctrl Pts',(-0.902193646979982,-0.237231147975234,
-1.3735491215176));
#29453=CARTESIAN_POINT('Ctrl Pts',(-0.920778333482564,-0.266264900654908,
-1.36127834356734));
#29454=CARTESIAN_POINT('Ctrl Pts',(-0.962485392528368,-0.317195968905306,
-1.33211611256184));
#29455=CARTESIAN_POINT('Ctrl Pts',(-0.985600426557816,-0.33909093068465,
-1.31521005565926));
#29456=CARTESIAN_POINT('Ctrl Pts',(-1.03253285680459,-0.373586846396559,
-1.27866649102984));
#29457=CARTESIAN_POINT('Ctrl Pts',(-1.05871835910697,-0.388086240756494,
-1.25722555095714));
#29458=CARTESIAN_POINT('Ctrl Pts',(-1.11153475808518,-0.407068917407805,
-1.2107812086231));
#29459=CARTESIAN_POINT('Ctrl Pts',(-1.13814686046673,-0.411552957311693,
-1.18575674747573));
#29460=CARTESIAN_POINT('Ctrl Pts',(-1.18575674747573,-0.411552957311693,
-1.13814686046673));
#29461=CARTESIAN_POINT('Ctrl Pts',(-1.2107812086231,-0.407068917407805,
-1.11153475808518));
#29462=CARTESIAN_POINT('Ctrl Pts',(-1.25722555095714,-0.388086240756494,
-1.05871835910697));
#29463=CARTESIAN_POINT('Ctrl Pts',(-1.27866649102984,-0.373586846396559,
-1.03253285680459));
#29464=CARTESIAN_POINT('Ctrl Pts',(-1.31521005565926,-0.33909093068465,
-0.985600426557816));
#29465=CARTESIAN_POINT('Ctrl Pts',(-1.33211611256184,-0.317195968905306,
-0.962485392528369));
#29466=CARTESIAN_POINT('Ctrl Pts',(-1.36127834356734,-0.266264900654909,
-0.920778333482565));
#29467=CARTESIAN_POINT('Ctrl Pts',(-1.3735491215176,-0.237231147975234,
-0.902193646979983));
#29468=CARTESIAN_POINT('Ctrl Pts',(-1.39550172959303,-0.166543350814306,
-0.867957148219442));
#29469=CARTESIAN_POINT('Ctrl Pts',(-1.40380622184538,-0.123401821157026,
-0.854205272175555));
#29470=CARTESIAN_POINT('Ctrl Pts',(-1.40825612658882,-0.07938,-0.846804978391753));
#29471=CARTESIAN_POINT('Origin',(-1.18440385848747,-0.07938,-1.18440385848747));
#29472=CARTESIAN_POINT('Origin',(0.,-0.07938,0.));
#29473=CARTESIAN_POINT('',(-0.397005914195118,-0.07938,-1.59456899932179));
#29474=CARTESIAN_POINT('Origin',(0.,-0.07938,0.));
#29475=CARTESIAN_POINT('Origin',(1.11022302462516E-16,-0.07938,-1.675));
#29476=CARTESIAN_POINT('Origin',(1.11022302462516E-16,0.,-1.675));
#29477=CARTESIAN_POINT('',(0.397005914195118,-0.07938,-1.59456899932179));
#29478=CARTESIAN_POINT('Ctrl Pts',(0.397005914195119,-0.0793800000000001,
-1.59456899932179));
#29479=CARTESIAN_POINT('Ctrl Pts',(0.388626558458099,-0.123401821157026,
-1.59665523941937));
#29480=CARTESIAN_POINT('Ctrl Pts',(0.373030350867485,-0.166543350814306,
-1.60050712143809));
#29481=CARTESIAN_POINT('Ctrl Pts',(0.333298652394954,-0.237231147975234,
-1.60919314384089));
#29482=CARTESIAN_POINT('Ctrl Pts',(0.311480544243686,-0.266264900654909,
-1.61365775139403));
#29483=CARTESIAN_POINT('Ctrl Pts',(0.261368388670537,-0.317195968905306,
-1.62252828437015));
#29484=CARTESIAN_POINT('Ctrl Pts',(0.233069203882014,-0.33909093068465,
-1.62691869420078));
#29485=CARTESIAN_POINT('Ctrl Pts',(0.174042761838763,-0.373586846396559,
-1.63426473152765));
#29486=CARTESIAN_POINT('Ctrl Pts',(0.140365781471549,-0.388086240756494,
-1.63761964365402));
#29487=CARTESIAN_POINT('Ctrl Pts',(0.0701778381840612,-0.407068917407805,
-1.64212536811722));
#29488=CARTESIAN_POINT('Ctrl Pts',(0.0336652739555916,-0.411552957311693,
-1.643248));
#29489=CARTESIAN_POINT('Ctrl Pts',(-0.0336652739555915,-0.411552957311693,
-1.643248));
#29490=CARTESIAN_POINT('Ctrl Pts',(-0.0701778381840612,-0.407068917407805,
-1.64212536811722));
#29491=CARTESIAN_POINT('Ctrl Pts',(-0.140365781471549,-0.388086240756494,
-1.63761964365402));
#29492=CARTESIAN_POINT('Ctrl Pts',(-0.174042761838764,-0.373586846396559,
-1.63426473152765));
#29493=CARTESIAN_POINT('Ctrl Pts',(-0.233069203882014,-0.33909093068465,
-1.62691869420078));
#29494=CARTESIAN_POINT('Ctrl Pts',(-0.261368388670536,-0.317195968905306,
-1.62252828437015));
#29495=CARTESIAN_POINT('Ctrl Pts',(-0.311480544243686,-0.266264900654908,
-1.61365775139403));
#29496=CARTESIAN_POINT('Ctrl Pts',(-0.333298652394954,-0.237231147975234,
-1.60919314384089));
#29497=CARTESIAN_POINT('Ctrl Pts',(-0.373030350867485,-0.166543350814306,
-1.60050712143809));
#29498=CARTESIAN_POINT('Ctrl Pts',(-0.388626558458099,-0.123401821157026,
-1.59665523941937));
#29499=CARTESIAN_POINT('Ctrl Pts',(-0.397005914195118,-0.07938,-1.59456899932179));
#29500=CARTESIAN_POINT('Origin',(1.11022302462516E-16,-0.07938,-1.675));
#29501=CARTESIAN_POINT('Origin',(0.,-0.07938,0.));
#29502=CARTESIAN_POINT('',(0.846804978391753,-0.07938,-1.40825612658882));
#29503=CARTESIAN_POINT('Origin',(0.,-0.07938,0.));
#29504=CARTESIAN_POINT('Origin',(1.18440385848747,-0.07938,-1.18440385848747));
#29505=CARTESIAN_POINT('Origin',(1.18440385848747,0.,-1.18440385848747));
#29506=CARTESIAN_POINT('',(1.40825612658882,-0.07938,-0.846804978391753));
#29507=CARTESIAN_POINT('Ctrl Pts',(1.40825612658882,-0.0793800000000001,
-0.846804978391753));
#29508=CARTESIAN_POINT('Ctrl Pts',(1.40380622184538,-0.123401821157026,
-0.854205272175555));
#29509=CARTESIAN_POINT('Ctrl Pts',(1.39550172959303,-0.166543350814306,
-0.867957148219442));
#29510=CARTESIAN_POINT('Ctrl Pts',(1.3735491215176,-0.237231147975234,-0.902193646979983));
#29511=CARTESIAN_POINT('Ctrl Pts',(1.36127834356734,-0.266264900654908,
-0.920778333482565));
#29512=CARTESIAN_POINT('Ctrl Pts',(1.33211611256184,-0.317195968905306,
-0.962485392528369));
#29513=CARTESIAN_POINT('Ctrl Pts',(1.31521005565926,-0.33909093068465,-0.985600426557816));
#29514=CARTESIAN_POINT('Ctrl Pts',(1.27866649102984,-0.373586846396559,
-1.03253285680459));
#29515=CARTESIAN_POINT('Ctrl Pts',(1.25722555095714,-0.388086240756494,
-1.05871835910697));
#29516=CARTESIAN_POINT('Ctrl Pts',(1.2107812086231,-0.407068917407805,-1.11153475808518));
#29517=CARTESIAN_POINT('Ctrl Pts',(1.18575674747573,-0.411552957311693,
-1.13814686046673));
#29518=CARTESIAN_POINT('Ctrl Pts',(1.13814686046673,-0.411552957311693,
-1.18575674747573));
#29519=CARTESIAN_POINT('Ctrl Pts',(1.11153475808518,-0.407068917407805,
-1.2107812086231));
#29520=CARTESIAN_POINT('Ctrl Pts',(1.05871835910697,-0.388086240756494,
-1.25722555095714));
#29521=CARTESIAN_POINT('Ctrl Pts',(1.03253285680459,-0.373586846396559,
-1.27866649102984));
#29522=CARTESIAN_POINT('Ctrl Pts',(0.985600426557816,-0.33909093068465,
-1.31521005565926));
#29523=CARTESIAN_POINT('Ctrl Pts',(0.962485392528369,-0.317195968905306,
-1.33211611256184));
#29524=CARTESIAN_POINT('Ctrl Pts',(0.920778333482565,-0.266264900654909,
-1.36127834356734));
#29525=CARTESIAN_POINT('Ctrl Pts',(0.902193646979983,-0.237231147975234,
-1.3735491215176));
#29526=CARTESIAN_POINT('Ctrl Pts',(0.867957148219442,-0.166543350814306,
-1.39550172959303));
#29527=CARTESIAN_POINT('Ctrl Pts',(0.854205272175555,-0.123401821157026,
-1.40380622184538));
#29528=CARTESIAN_POINT('Ctrl Pts',(0.846804978391753,-0.0793800000000001,
-1.40825612658882));
#29529=CARTESIAN_POINT('Origin',(1.18440385848747,-0.07938,-1.18440385848747));
#29530=CARTESIAN_POINT('Origin',(0.,-0.27783,0.));
#29531=CARTESIAN_POINT('',(-1.643248,-0.47628,2.01239840340529E-16));
#29532=CARTESIAN_POINT('Origin',(0.,-0.47628,0.));
#29533=CARTESIAN_POINT('',(-1.643248,-0.27783,2.01239840340529E-16));
#29534=CARTESIAN_POINT('',(1.59456899932179,-0.07938,0.397005914195118));
#29535=CARTESIAN_POINT('Origin',(0.,-0.07938,0.));
#29536=CARTESIAN_POINT('',(1.59456899932179,-0.07938,-0.397005914195118));
#29537=CARTESIAN_POINT('Ctrl Pts',(1.59456899932179,-0.0793800000000001,
0.397005914195118));
#29538=CARTESIAN_POINT('Ctrl Pts',(1.59665523941937,-0.123401821157026,
0.388626558458099));
#29539=CARTESIAN_POINT('Ctrl Pts',(1.60050712143809,-0.166543350814306,
0.373030350867485));
#29540=CARTESIAN_POINT('Ctrl Pts',(1.60919314384089,-0.237231147975234,
0.333298652394954));
#29541=CARTESIAN_POINT('Ctrl Pts',(1.61365775139403,-0.266264900654909,
0.311480544243686));
#29542=CARTESIAN_POINT('Ctrl Pts',(1.62252828437015,-0.317195968905306,
0.261368388670537));
#29543=CARTESIAN_POINT('Ctrl Pts',(1.62691869420078,-0.33909093068465,0.233069203882014));
#29544=CARTESIAN_POINT('Ctrl Pts',(1.63426473152765,-0.373586846396559,
0.174042761838764));
#29545=CARTESIAN_POINT('Ctrl Pts',(1.63761964365402,-0.388086240756494,
0.140365781471549));
#29546=CARTESIAN_POINT('Ctrl Pts',(1.64212536811722,-0.407068917407805,
0.0701778381840612));
#29547=CARTESIAN_POINT('Ctrl Pts',(1.643248,-0.411552957311693,0.0336652739555916));
#29548=CARTESIAN_POINT('Ctrl Pts',(1.643248,-0.411552957311693,-0.0336652739555916));
#29549=CARTESIAN_POINT('Ctrl Pts',(1.64212536811722,-0.407068917407805,
-0.0701778381840612));
#29550=CARTESIAN_POINT('Ctrl Pts',(1.63761964365402,-0.388086240756494,
-0.140365781471549));
#29551=CARTESIAN_POINT('Ctrl Pts',(1.63426473152765,-0.373586846396559,
-0.174042761838764));
#29552=CARTESIAN_POINT('Ctrl Pts',(1.62691869420078,-0.33909093068465,-0.233069203882014));
#29553=CARTESIAN_POINT('Ctrl Pts',(1.62252828437015,-0.317195968905306,
-0.261368388670537));
#29554=CARTESIAN_POINT('Ctrl Pts',(1.61365775139403,-0.266264900654909,
-0.311480544243686));
#29555=CARTESIAN_POINT('Ctrl Pts',(1.60919314384089,-0.237231147975234,
-0.333298652394954));
#29556=CARTESIAN_POINT('Ctrl Pts',(1.60050712143809,-0.166543350814306,
-0.373030350867485));
#29557=CARTESIAN_POINT('Ctrl Pts',(1.59665523941937,-0.123401821157026,
-0.388626558458099));
#29558=CARTESIAN_POINT('Ctrl Pts',(1.59456899932179,-0.07938,-0.397005914195118));
#29559=CARTESIAN_POINT('Origin',(0.,-0.07938,0.));
#29560=CARTESIAN_POINT('Origin',(0.,-0.07938,0.));
#29561=CARTESIAN_POINT('Origin',(1.675,-0.07938,0.));
#29562=CARTESIAN_POINT('Origin',(1.675,0.,0.));
#29563=CARTESIAN_POINT('Origin',(1.675,-0.07938,0.));
#29564=CARTESIAN_POINT('Origin',(0.,-0.47628,0.));
#29565=CARTESIAN_POINT('Origin',(0.,-0.07938,0.));
#43421=UNCERTAINTY_MEASURE_WITH_UNIT(LENGTH_MEASURE(0.001),#43522,
'DISTANCE_ACCURACY_VALUE',
'Maximum model space distance between geometric entities at asserted c
onnectivities');
#43453=UNCERTAINTY_MEASURE_WITH_UNIT(LENGTH_MEASURE(0.001),#43522,
'DISTANCE_ACCURACY_VALUE',
'Maximum model space distance between geometric entities at asserted c
onnectivities');
#43489=(
GEOMETRIC_REPRESENTATION_CONTEXT(3)
GLOBAL_UNCERTAINTY_ASSIGNED_CONTEXT((#43421))
GLOBAL_UNIT_ASSIGNED_CONTEXT((#43522,#43524,#43525))
REPRESENTATION_CONTEXT('','3D')
);
#43521=(
GEOMETRIC_REPRESENTATION_CONTEXT(3)
GLOBAL_UNCERTAINTY_ASSIGNED_CONTEXT((#43453))
GLOBAL_UNIT_ASSIGNED_CONTEXT((#43522,#43524,#43525))
REPRESENTATION_CONTEXT('','3D')
);
#43522=(
LENGTH_UNIT()
NAMED_UNIT(*)
SI_UNIT(.CENTI.,.METRE.)
);
#43524=(
NAMED_UNIT(*)
PLANE_ANGLE_UNIT()
SI_UNIT($,.RADIAN.)
);
#43525=(
NAMED_UNIT(*)
SI_UNIT($,.STERADIAN.)
SOLID_ANGLE_UNIT()
);
#43561=SHAPE_DEFINITION_REPRESENTATION(#43633,#43829);
#43633=PRODUCT_DEFINITION_SHAPE('',$,#43897);
#43829=SHAPE_REPRESENTATION('',(#20178),#43489);
#43861=PRODUCT_DEFINITION_CONTEXT('part definition',#44064,'design');
#43897=PRODUCT_DEFINITION('Cage (1)','Cage (1)',#43964,#43861);
#43964=PRODUCT_DEFINITION_FORMATION('',$,#44101);
#44064=APPLICATION_CONTEXT(
'Core Data for Automotive Mechanical Design Process');
#44065=PRODUCT_CONTEXT('part definition',#44064,'mechanical');
#44101=PRODUCT('Cage (1)','Cage (1)','Cage (1)',(#44065));
#44196=COLOUR_RGB('Grey',0.48,0.52,0.57);
#44197=FILL_AREA_STYLE_COLOUR('',#44196);
#44198=FILL_AREA_STYLE('',(#44197));
#44199=SURFACE_STYLE_FILL_AREA(#44198);
#44200=SURFACE_SIDE_STYLE('',(#44199));
#44201=SURFACE_STYLE_USAGE(.BOTH.,#44200);
#44202=PRESENTATION_STYLE_ASSIGNMENT((#44201));
ENDSEC;
END-ISO-10303-21;
